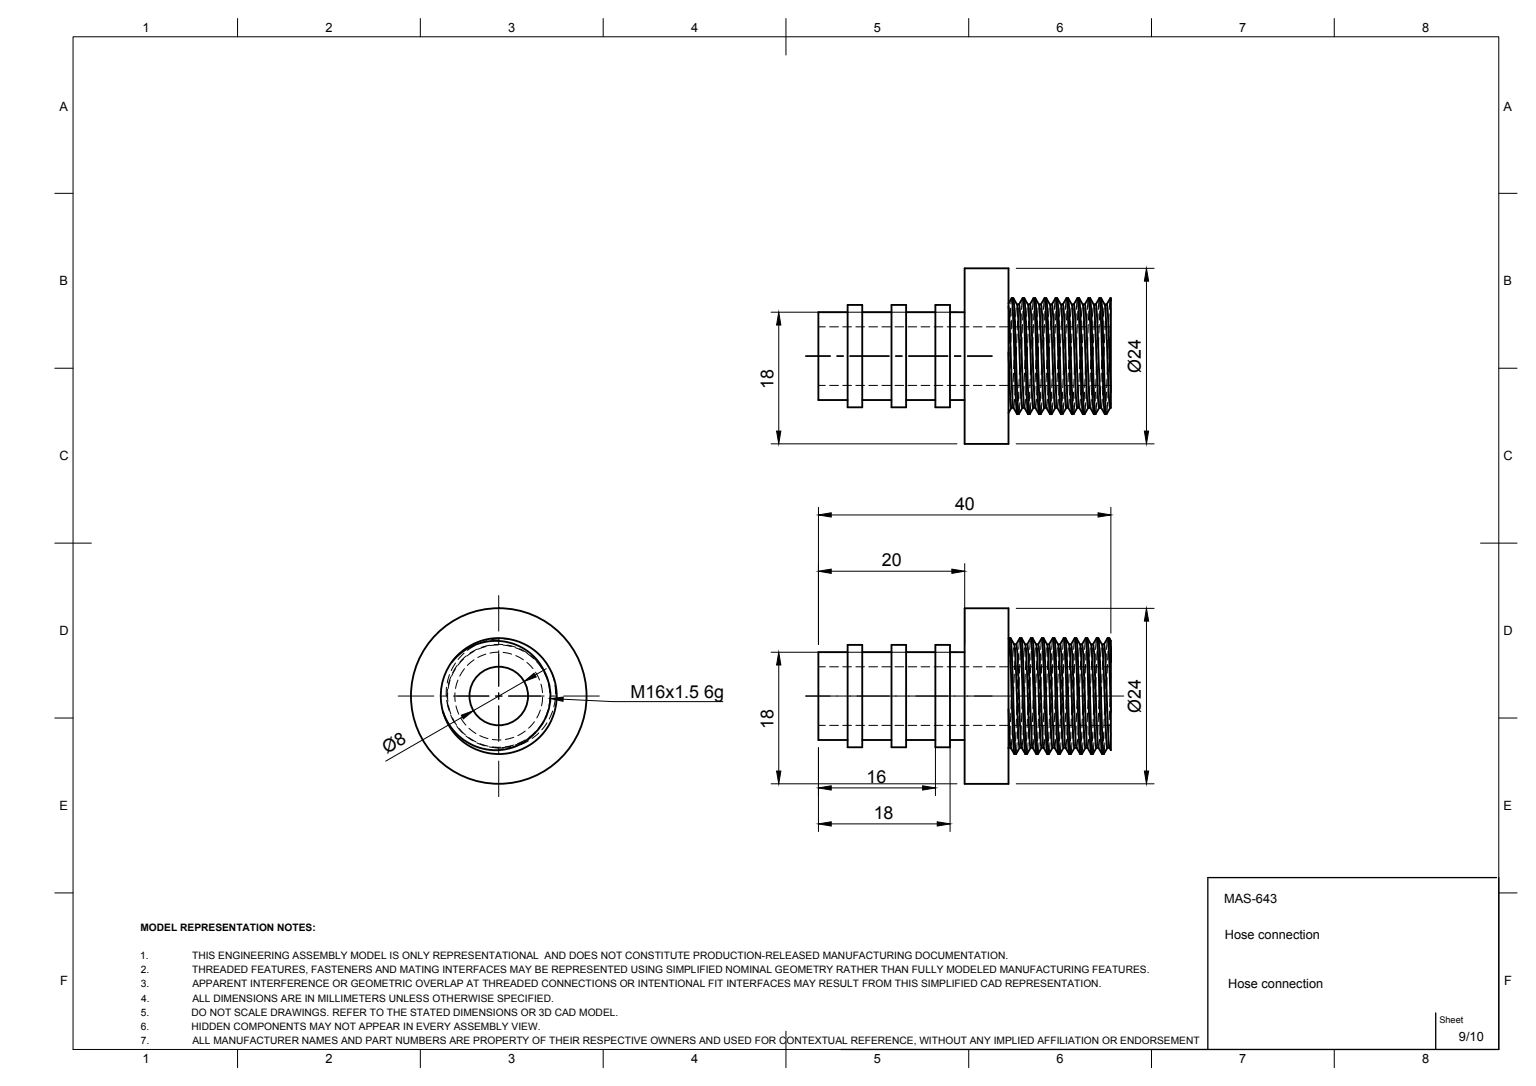
ISO-10303-21;
HEADER;
/* Generated by software containing ST-Developer
 * from STEP Tools, Inc. (www.steptools.com) 
 */

FILE_DESCRIPTION(
/* description */ ('Independent eighteen-tube parallel-flow evaporator geometry. Repeated
 machined headers and gasketed service covers, eighteen copper tubes, 
twenty-nine punched fins, threaded hose connections and bolted mountin
g feet. Native editable features and instanced parts. Braze details, w
orking fluid, pressure and thermal ratings require engineering selecti
on.'),
/* implementation_level */ '2;1');

FILE_NAME(
/* name */ 'Hose connection.step',
/* time_stamp */ '2026-11-08T20:53:59-08:00',
/* author */ (''),
/* organization */ (''),
/* preprocessor_version */ 'ST-DEVELOPER v20.2',
/* originating_system */ 'Autodesk Translation Framework v15.17.0.0',
/* authorisation */ '');

FILE_SCHEMA (('AUTOMOTIVE_DESIGN { 1 0 10303 214 3 1 1 }'));
ENDSEC;

DATA;
#10=MECHANICAL_DESIGN_GEOMETRIC_PRESENTATION_REPRESENTATION('',(#341),#42620);
#321=SHAPE_REPRESENTATION_RELATIONSHIP('SRR','None',#42731,#331);
#331=ADVANCED_BREP_SHAPE_REPRESENTATION('',(#351),#42618);
#341=STYLED_ITEM('',(#42787),#351);
#351=MANIFOLD_SOLID_BREP('Body1',#10391);
#475=FACE_BOUND('',#1791,.T.);
#476=FACE_BOUND('',#1793,.T.);
#477=FACE_BOUND('',#1797,.T.);
#478=FACE_BOUND('',#1799,.T.);
#479=FACE_BOUND('',#1803,.T.);
#480=FACE_BOUND('',#1805,.T.);
#481=FACE_BOUND('',#1810,.T.);
#482=FACE_BOUND('',#1812,.T.);
#483=FACE_BOUND('',#1815,.T.);
#484=FACE_BOUND('',#1818,.T.);
#567=PLANE('',#11185);
#568=PLANE('',#11188);
#569=PLANE('',#11194);
#570=PLANE('',#11196);
#571=PLANE('',#11202);
#572=PLANE('',#11204);
#573=PLANE('',#11212);
#574=PLANE('',#11214);
#575=PLANE('',#11218);
#576=PLANE('',#11221);
#601=B_SPLINE_SURFACE_WITH_KNOTS('',3,3,((#40929,#40930,#40931,#40932,#40933,
#40934,#40935,#40936,#40937,#40938,#40939,#40940,#40941,#40942,#40943,#40944,
#40945,#40946,#40947,#40948,#40949,#40950,#40951,#40952,#40953,#40954,#40955,
#40956,#40957,#40958,#40959,#40960,#40961,#40962,#40963,#40964,#40965,#40966,
#40967,#40968,#40969,#40970,#40971,#40972,#40973,#40974,#40975,#40976,#40977,
#40978,#40979,#40980,#40981,#40982,#40983,#40984,#40985,#40986,#40987,#40988,
#40989,#40990,#40991,#40992,#40993,#40994,#40995,#40996,#40997,#40998,#40999,
#41000,#41001,#41002,#41003,#41004,#41005,#41006,#41007,#41008,#41009,#41010,
#41011,#41012,#41013,#41014,#41015,#41016,#41017,#41018,#41019,#41020,#41021,
#41022,#41023,#41024,#41025,#41026,#41027,#41028,#41029,#41030,#41031,#41032,
#41033,#41034,#41035,#41036,#41037,#41038,#41039,#41040,#41041,#41042,#41043,
#41044,#41045,#41046,#41047,#41048,#41049,#41050,#41051,#41052,#41053),
(#41054,#41055,#41056,#41057,#41058,#41059,#41060,#41061,#41062,#41063,
#41064,#41065,#41066,#41067,#41068,#41069,#41070,#41071,#41072,#41073,#41074,
#41075,#41076,#41077,#41078,#41079,#41080,#41081,#41082,#41083,#41084,#41085,
#41086,#41087,#41088,#41089,#41090,#41091,#41092,#41093,#41094,#41095,#41096,
#41097,#41098,#41099,#41100,#41101,#41102,#41103,#41104,#41105,#41106,#41107,
#41108,#41109,#41110,#41111,#41112,#41113,#41114,#41115,#41116,#41117,#41118,
#41119,#41120,#41121,#41122,#41123,#41124,#41125,#41126,#41127,#41128,#41129,
#41130,#41131,#41132,#41133,#41134,#41135,#41136,#41137,#41138,#41139,#41140,
#41141,#41142,#41143,#41144,#41145,#41146,#41147,#41148,#41149,#41150,#41151,
#41152,#41153,#41154,#41155,#41156,#41157,#41158,#41159,#41160,#41161,#41162,
#41163,#41164,#41165,#41166,#41167,#41168,#41169,#41170,#41171,#41172,#41173,
#41174,#41175,#41176,#41177,#41178),(#41179,#41180,#41181,#41182,#41183,
#41184,#41185,#41186,#41187,#41188,#41189,#41190,#41191,#41192,#41193,#41194,
#41195,#41196,#41197,#41198,#41199,#41200,#41201,#41202,#41203,#41204,#41205,
#41206,#41207,#41208,#41209,#41210,#41211,#41212,#41213,#41214,#41215,#41216,
#41217,#41218,#41219,#41220,#41221,#41222,#41223,#41224,#41225,#41226,#41227,
#41228,#41229,#41230,#41231,#41232,#41233,#41234,#41235,#41236,#41237,#41238,
#41239,#41240,#41241,#41242,#41243,#41244,#41245,#41246,#41247,#41248,#41249,
#41250,#41251,#41252,#41253,#41254,#41255,#41256,#41257,#41258,#41259,#41260,
#41261,#41262,#41263,#41264,#41265,#41266,#41267,#41268,#41269,#41270,#41271,
#41272,#41273,#41274,#41275,#41276,#41277,#41278,#41279,#41280,#41281,#41282,
#41283,#41284,#41285,#41286,#41287,#41288,#41289,#41290,#41291,#41292,#41293,
#41294,#41295,#41296,#41297,#41298,#41299,#41300,#41301,#41302,#41303),
(#41304,#41305,#41306,#41307,#41308,#41309,#41310,#41311,#41312,#41313,
#41314,#41315,#41316,#41317,#41318,#41319,#41320,#41321,#41322,#41323,#41324,
#41325,#41326,#41327,#41328,#41329,#41330,#41331,#41332,#41333,#41334,#41335,
#41336,#41337,#41338,#41339,#41340,#41341,#41342,#41343,#41344,#41345,#41346,
#41347,#41348,#41349,#41350,#41351,#41352,#41353,#41354,#41355,#41356,#41357,
#41358,#41359,#41360,#41361,#41362,#41363,#41364,#41365,#41366,#41367,#41368,
#41369,#41370,#41371,#41372,#41373,#41374,#41375,#41376,#41377,#41378,#41379,
#41380,#41381,#41382,#41383,#41384,#41385,#41386,#41387,#41388,#41389,#41390,
#41391,#41392,#41393,#41394,#41395,#41396,#41397,#41398,#41399,#41400,#41401,
#41402,#41403,#41404,#41405,#41406,#41407,#41408,#41409,#41410,#41411,#41412,
#41413,#41414,#41415,#41416,#41417,#41418,#41419,#41420,#41421,#41422,#41423,
#41424,#41425,#41426,#41427,#41428)),.UNSPECIFIED.,.F.,.F.,.F.,(4,4),(4,
1,1,1,1,1,1,1,1,1,1,1,1,1,1,1,1,1,1,1,1,1,1,1,1,1,1,1,1,1,1,1,1,1,1,1,1,
1,1,1,1,1,1,1,1,1,1,1,1,1,1,1,1,1,1,1,1,1,1,1,1,1,1,1,1,1,1,1,1,1,1,1,1,
1,1,1,1,1,1,1,1,1,1,1,1,1,1,1,1,1,1,1,1,1,1,1,1,1,1,1,1,1,1,1,1,1,1,1,1,
1,1,1,1,1,1,1,1,1,1,1,1,1,4),(0.,0.0989001011121828),(8.30505915324874,
8.80271834784681,9.30037754244489,9.79803673704296,10.295695931641,10.7933551262391,
11.2910143208372,11.7886735154353,12.2863327100333,12.7839919046314,13.2816510992295,
13.7793102938275,14.2769694884256,14.7746286830237,15.2722878776218,15.7699470722198,
16.2676062668179,16.765265461416,17.2629246560141,17.7605838506121,18.2582430452102,
18.7559022398083,19.2535614344064,19.7512206290044,20.2488798236025,20.7465390182006,
21.2441982127987,21.7418574073967,22.2395166019948,22.7371757965929,23.2348349911909,
23.732494185789,24.2301533803871,24.7278125749852,25.2254717695832,25.7231309641813,
26.2207901587794,26.7184493533775,27.2161085479755,27.7137677425736,28.2114269371717,
28.7090861317698,29.2067453263678,29.7044045209659,30.202063715564,30.699722910162,
31.1973821047601,31.6950412993582,32.1927004939563,32.6903596885543,33.1880188831524,
33.6856780777505,34.1833372723486,34.6809964669466,35.1786556615447,35.6763148561428,
36.1739740507409,36.6716332453389,37.169292439937,37.6669516345351,38.1646108291331,
38.6622700237312,39.1599292183293,39.6575884129274,40.1552476075254,40.6529068021235,
41.1505659967216,41.6482251913197,42.1458843859177,42.6435435805158,43.1412027751139,
43.638861969712,44.13652116431,44.6341803589081,45.1318395535062,45.6294987481042,
46.1271579427023,46.6248171373004,47.1224763318985,47.6201355264965,48.1177947210946,
48.6154539156927,49.1131131102908,49.6107723048888,50.1084314994869,50.606090694085,
51.103749888683,51.6014090832811,52.0990682778792,52.5967274724773,53.0943866670753,
53.5920458616734,54.0897050562715,54.5873642508696,55.0850234454676,55.5826826400657,
56.0803418346638,56.5780010292619,57.0756602238599,57.573319418458,58.0709786130561,
58.5686378076541,59.0662970022522,59.5639561968503,60.0616153914484,60.5592745860464,
61.0569337806445,61.5545929752426,62.0522521698407,62.5499113644387,63.0475705590368,
63.5452297536349,64.042888948233,64.540548142831,65.0382073374291,65.5358665320272,
66.0335257266252,66.5311849212233,67.0288441158214,67.5265033104195,68.0241625050175,
68.5218216996156,69.0194808942137),.UNSPECIFIED.);
#602=B_SPLINE_SURFACE_WITH_KNOTS('',3,3,((#41703,#41704,#41705,#41706,#41707,
#41708,#41709,#41710,#41711,#41712,#41713,#41714,#41715,#41716,#41717,#41718,
#41719,#41720,#41721,#41722,#41723,#41724,#41725,#41726,#41727,#41728,#41729,
#41730,#41731,#41732,#41733,#41734,#41735,#41736,#41737,#41738,#41739,#41740,
#41741,#41742,#41743,#41744,#41745,#41746,#41747,#41748,#41749,#41750,#41751,
#41752,#41753,#41754,#41755,#41756,#41757,#41758,#41759,#41760,#41761,#41762,
#41763,#41764,#41765,#41766,#41767,#41768,#41769,#41770,#41771,#41772,#41773,
#41774,#41775,#41776,#41777,#41778,#41779,#41780,#41781,#41782,#41783,#41784,
#41785,#41786,#41787,#41788,#41789,#41790,#41791,#41792,#41793,#41794,#41795,
#41796,#41797,#41798,#41799,#41800,#41801,#41802,#41803,#41804,#41805,#41806,
#41807,#41808,#41809,#41810,#41811,#41812,#41813,#41814,#41815,#41816,#41817,
#41818,#41819,#41820,#41821,#41822,#41823,#41824,#41825,#41826,#41827),
(#41828,#41829,#41830,#41831,#41832,#41833,#41834,#41835,#41836,#41837,
#41838,#41839,#41840,#41841,#41842,#41843,#41844,#41845,#41846,#41847,#41848,
#41849,#41850,#41851,#41852,#41853,#41854,#41855,#41856,#41857,#41858,#41859,
#41860,#41861,#41862,#41863,#41864,#41865,#41866,#41867,#41868,#41869,#41870,
#41871,#41872,#41873,#41874,#41875,#41876,#41877,#41878,#41879,#41880,#41881,
#41882,#41883,#41884,#41885,#41886,#41887,#41888,#41889,#41890,#41891,#41892,
#41893,#41894,#41895,#41896,#41897,#41898,#41899,#41900,#41901,#41902,#41903,
#41904,#41905,#41906,#41907,#41908,#41909,#41910,#41911,#41912,#41913,#41914,
#41915,#41916,#41917,#41918,#41919,#41920,#41921,#41922,#41923,#41924,#41925,
#41926,#41927,#41928,#41929,#41930,#41931,#41932,#41933,#41934,#41935,#41936,
#41937,#41938,#41939,#41940,#41941,#41942,#41943,#41944,#41945,#41946,#41947,
#41948,#41949,#41950,#41951,#41952),(#41953,#41954,#41955,#41956,#41957,
#41958,#41959,#41960,#41961,#41962,#41963,#41964,#41965,#41966,#41967,#41968,
#41969,#41970,#41971,#41972,#41973,#41974,#41975,#41976,#41977,#41978,#41979,
#41980,#41981,#41982,#41983,#41984,#41985,#41986,#41987,#41988,#41989,#41990,
#41991,#41992,#41993,#41994,#41995,#41996,#41997,#41998,#41999,#42000,#42001,
#42002,#42003,#42004,#42005,#42006,#42007,#42008,#42009,#42010,#42011,#42012,
#42013,#42014,#42015,#42016,#42017,#42018,#42019,#42020,#42021,#42022,#42023,
#42024,#42025,#42026,#42027,#42028,#42029,#42030,#42031,#42032,#42033,#42034,
#42035,#42036,#42037,#42038,#42039,#42040,#42041,#42042,#42043,#42044,#42045,
#42046,#42047,#42048,#42049,#42050,#42051,#42052,#42053,#42054,#42055,#42056,
#42057,#42058,#42059,#42060,#42061,#42062,#42063,#42064,#42065,#42066,#42067,
#42068,#42069,#42070,#42071,#42072,#42073,#42074,#42075,#42076,#42077),
(#42078,#42079,#42080,#42081,#42082,#42083,#42084,#42085,#42086,#42087,
#42088,#42089,#42090,#42091,#42092,#42093,#42094,#42095,#42096,#42097,#42098,
#42099,#42100,#42101,#42102,#42103,#42104,#42105,#42106,#42107,#42108,#42109,
#42110,#42111,#42112,#42113,#42114,#42115,#42116,#42117,#42118,#42119,#42120,
#42121,#42122,#42123,#42124,#42125,#42126,#42127,#42128,#42129,#42130,#42131,
#42132,#42133,#42134,#42135,#42136,#42137,#42138,#42139,#42140,#42141,#42142,
#42143,#42144,#42145,#42146,#42147,#42148,#42149,#42150,#42151,#42152,#42153,
#42154,#42155,#42156,#42157,#42158,#42159,#42160,#42161,#42162,#42163,#42164,
#42165,#42166,#42167,#42168,#42169,#42170,#42171,#42172,#42173,#42174,#42175,
#42176,#42177,#42178,#42179,#42180,#42181,#42182,#42183,#42184,#42185,#42186,
#42187,#42188,#42189,#42190,#42191,#42192,#42193,#42194,#42195,#42196,#42197,
#42198,#42199,#42200,#42201,#42202)),.UNSPECIFIED.,.F.,.F.,.F.,(4,4),(4,
1,1,1,1,1,1,1,1,1,1,1,1,1,1,1,1,1,1,1,1,1,1,1,1,1,1,1,1,1,1,1,1,1,1,1,1,
1,1,1,1,1,1,1,1,1,1,1,1,1,1,1,1,1,1,1,1,1,1,1,1,1,1,1,1,1,1,1,1,1,1,1,1,
1,1,1,1,1,1,1,1,1,1,1,1,1,1,1,1,1,1,1,1,1,1,1,1,1,1,1,1,1,1,1,1,1,1,1,1,
1,1,1,1,1,1,1,1,1,1,1,1,1,4),(0.,0.0989001011121828),(11.6147305479242,
12.1123897425223,12.6100489371204,13.1077081317185,13.6053673263165,14.1030265209146,
14.6006857155127,15.0983449101107,15.5960041047088,16.0936632993069,16.591322493905,
17.088981688503,17.5866408831011,18.0843000776992,18.5819592722973,19.0796184668953,
19.5772776614934,20.0749368560915,20.5725960506896,21.0702552452876,21.5679144398857,
22.0655736344838,22.5632328290818,23.0608920236799,23.558551218278,24.0562104128761,
24.5538696074741,25.0515288020722,25.5491879966703,26.0468471912684,26.5445063858664,
27.0421655804645,27.5398247750626,28.0374839696607,28.5351431642587,29.0328023588568,
29.5304615534549,30.0281207480529,30.525779942651,31.0234391372491,31.5210983318472,
32.0187575264452,32.5164167210433,33.0140759156414,33.5117351102395,34.0093943048375,
34.5070534994356,35.0047126940337,35.5023718886318,36.0000310832298,36.4976902778279,
36.995349472426,37.4930086670241,37.9906678616221,38.4883270562202,38.9859862508183,
39.4836454454163,39.9813046400144,40.4789638346125,40.9766230292106,41.4742822238086,
41.9719414184067,42.4696006130048,42.9672598076029,43.4649190022009,43.962578196799,
44.4602373913971,44.9578965859952,45.4555557805932,45.9532149751913,46.4508741697894,
46.9485333643874,47.4461925589855,47.9438517535836,48.4415109481817,48.9391701427797,
49.4368293373778,49.9344885319759,50.432147726574,50.929806921172,51.4274661157701,
51.9251253103682,52.4227845049663,52.9204436995643,53.4181028941624,53.9157620887605,
54.4134212833585,54.9110804779566,55.4087396725547,55.9063988671528,56.4040580617508,
56.9017172563489,57.399376450947,57.8970356455451,58.3946948401431,58.8923540347412,
59.3900132293393,59.8876724239374,60.3853316185354,60.8829908131335,61.3806500077316,
61.8783092023296,62.3759683969277,62.8736275915258,63.3712867861239,63.8689459807219,
64.36660517532,64.8642643699181,65.3619235645162,65.8595827591142,66.3572419537123,
66.8549011483104,67.3525603429085,67.8502195375065,68.3478787321046,68.8455379267027,
69.3431971213007,69.8408563158988,70.3385155104969,70.836174705095,71.333833899693,
71.8314930942911,72.3291522888892),.UNSPECIFIED.);
#1101=FACE_OUTER_BOUND('',#1767,.T.);
#1102=FACE_OUTER_BOUND('',#1768,.T.);
#1103=FACE_OUTER_BOUND('',#1769,.T.);
#1104=FACE_OUTER_BOUND('',#1770,.T.);
#1105=FACE_OUTER_BOUND('',#1771,.T.);
#1106=FACE_OUTER_BOUND('',#1772,.T.);
#1107=FACE_OUTER_BOUND('',#1773,.T.);
#1108=FACE_OUTER_BOUND('',#1774,.T.);
#1109=FACE_OUTER_BOUND('',#1775,.T.);
#1110=FACE_OUTER_BOUND('',#1776,.T.);
#1111=FACE_OUTER_BOUND('',#1777,.T.);
#1112=FACE_OUTER_BOUND('',#1778,.T.);
#1113=FACE_OUTER_BOUND('',#1779,.T.);
#1114=FACE_OUTER_BOUND('',#1780,.T.);
#1115=FACE_OUTER_BOUND('',#1781,.T.);
#1116=FACE_OUTER_BOUND('',#1782,.T.);
#1117=FACE_OUTER_BOUND('',#1783,.T.);
#1118=FACE_OUTER_BOUND('',#1784,.T.);
#1119=FACE_OUTER_BOUND('',#1785,.T.);
#1120=FACE_OUTER_BOUND('',#1786,.T.);
#1121=FACE_OUTER_BOUND('',#1787,.T.);
#1122=FACE_OUTER_BOUND('',#1788,.T.);
#1123=FACE_OUTER_BOUND('',#1789,.T.);
#1124=FACE_OUTER_BOUND('',#1790,.T.);
#1125=FACE_OUTER_BOUND('',#1792,.T.);
#1126=FACE_OUTER_BOUND('',#1794,.T.);
#1127=FACE_OUTER_BOUND('',#1795,.T.);
#1128=FACE_OUTER_BOUND('',#1796,.T.);
#1129=FACE_OUTER_BOUND('',#1798,.T.);
#1130=FACE_OUTER_BOUND('',#1800,.T.);
#1131=FACE_OUTER_BOUND('',#1801,.T.);
#1132=FACE_OUTER_BOUND('',#1802,.T.);
#1133=FACE_OUTER_BOUND('',#1804,.T.);
#1134=FACE_OUTER_BOUND('',#1806,.T.);
#1135=FACE_OUTER_BOUND('',#1807,.T.);
#1136=FACE_OUTER_BOUND('',#1808,.T.);
#1137=FACE_OUTER_BOUND('',#1809,.T.);
#1138=FACE_OUTER_BOUND('',#1811,.T.);
#1139=FACE_OUTER_BOUND('',#1813,.T.);
#1140=FACE_OUTER_BOUND('',#1814,.T.);
#1141=FACE_OUTER_BOUND('',#1816,.T.);
#1142=FACE_OUTER_BOUND('',#1817,.T.);
#1767=EDGE_LOOP('',(#9209,#9210,#9211,#9212));
#1768=EDGE_LOOP('',(#9213,#9214,#9215,#9216));
#1769=EDGE_LOOP('',(#9217,#9218,#9219,#9220));
#1770=EDGE_LOOP('',(#9221,#9222,#9223,#9224));
#1771=EDGE_LOOP('',(#9225,#9226,#9227,#9228));
#1772=EDGE_LOOP('',(#9229,#9230,#9231,#9232));
#1773=EDGE_LOOP('',(#9233,#9234,#9235,#9236));
#1774=EDGE_LOOP('',(#9237,#9238,#9239,#9240));
#1775=EDGE_LOOP('',(#9241,#9242,#9243,#9244));
#1776=EDGE_LOOP('',(#9245,#9246,#9247,#9248));
#1777=EDGE_LOOP('',(#9249,#9250,#9251,#9252));
#1778=EDGE_LOOP('',(#9253,#9254,#9255,#9256));
#1779=EDGE_LOOP('',(#9257,#9258,#9259,#9260));
#1780=EDGE_LOOP('',(#9261,#9262,#9263,#9264));
#1781=EDGE_LOOP('',(#9265,#9266,#9267,#9268));
#1782=EDGE_LOOP('',(#9269,#9270,#9271,#9272));
#1783=EDGE_LOOP('',(#9273,#9274,#9275,#9276));
#1784=EDGE_LOOP('',(#9277,#9278,#9279,#9280));
#1785=EDGE_LOOP('',(#9281,#9282,#9283,#9284));
#1786=EDGE_LOOP('',(#9285,#9286,#9287,#9288,#9289,#9290,#9291,#9292,#9293,
#9294,#9295,#9296,#9297,#9298,#9299,#9300,#9301,#9302,#9303,#9304,#9305,
#9306,#9307));
#1787=EDGE_LOOP('',(#9308,#9309,#9310,#9311));
#1788=EDGE_LOOP('',(#9312,#9313,#9314,#9315,#9316,#9317,#9318,#9319,#9320,
#9321,#9322,#9323,#9324,#9325,#9326,#9327,#9328,#9329,#9330,#9331,#9332,
#9333,#9334));
#1789=EDGE_LOOP('',(#9335,#9336,#9337,#9338));
#1790=EDGE_LOOP('',(#9339));
#1791=EDGE_LOOP('',(#9340));
#1792=EDGE_LOOP('',(#9341));
#1793=EDGE_LOOP('',(#9342));
#1794=EDGE_LOOP('',(#9343,#9344,#9345,#9346));
#1795=EDGE_LOOP('',(#9347,#9348,#9349,#9350));
#1796=EDGE_LOOP('',(#9351));
#1797=EDGE_LOOP('',(#9352));
#1798=EDGE_LOOP('',(#9353));
#1799=EDGE_LOOP('',(#9354));
#1800=EDGE_LOOP('',(#9355,#9356,#9357,#9358));
#1801=EDGE_LOOP('',(#9359,#9360,#9361,#9362));
#1802=EDGE_LOOP('',(#9363));
#1803=EDGE_LOOP('',(#9364));
#1804=EDGE_LOOP('',(#9365));
#1805=EDGE_LOOP('',(#9366));
#1806=EDGE_LOOP('',(#9367,#9368,#9369,#9370));
#1807=EDGE_LOOP('',(#9371,#9372,#9373,#9374));
#1808=EDGE_LOOP('',(#9375,#9376,#9377,#9378));
#1809=EDGE_LOOP('',(#9379));
#1810=EDGE_LOOP('',(#9380));
#1811=EDGE_LOOP('',(#9381));
#1812=EDGE_LOOP('',(#9382,#9383,#9384,#9385));
#1813=EDGE_LOOP('',(#9386,#9387,#9388,#9389));
#1814=EDGE_LOOP('',(#9390));
#1815=EDGE_LOOP('',(#9391));
#1816=EDGE_LOOP('',(#9392,#9393,#9394,#9395));
#1817=EDGE_LOOP('',(#9396,#9397,#9398,#9399));
#1818=EDGE_LOOP('',(#9400));
#1995=CIRCLE('',#11161,7.925);
#1996=CIRCLE('',#11172,7.0685);
#1997=CIRCLE('',#11182,7.0685);
#1998=CIRCLE('',#11184,7.925);
#1999=CIRCLE('',#11186,7.);
#2000=CIRCLE('',#11187,6.);
#2001=CIRCLE('',#11189,7.);
#2002=CIRCLE('',#11190,6.);
#2003=CIRCLE('',#11193,6.);
#2004=CIRCLE('',#11195,7.);
#2005=CIRCLE('',#11197,7.);
#2006=CIRCLE('',#11198,6.);
#2007=CIRCLE('',#11201,6.);
#2008=CIRCLE('',#11203,7.);
#2009=CIRCLE('',#11205,7.);
#2010=CIRCLE('',#11206,6.);
#2011=CIRCLE('',#11209,6.);
#2012=CIRCLE('',#11211,6.);
#2013=CIRCLE('',#11213,4.);
#2014=CIRCLE('',#11215,12.);
#2015=CIRCLE('',#11217,12.);
#2016=CIRCLE('',#11220,4.);
#2753=B_SPLINE_CURVE_WITH_KNOTS('',3,(#39788,#39789,#39790,#39791,#39792,
#39793,#39794,#39795,#39796,#39797,#39798,#39799,#39800,#39801,#39802,#39803),
 .UNSPECIFIED.,.F.,.F.,(4,3,3,3,3,4),(-4.09323272002468,-3.98127355678459,
-3.48361436218651,-2.98595516758844,-2.48829597299037,-2.07135887395548),
 .UNSPECIFIED.);
#2754=B_SPLINE_CURVE_WITH_KNOTS('',3,(#39806,#39807,#39808,#39809,#39810,
#39811,#39812,#39813,#39814,#39815),.UNSPECIFIED.,.F.,.F.,(4,3,3,4),(0.,
0.497659194598067,0.995318389196143,1.11971880752056),.UNSPECIFIED.);
#2755=B_SPLINE_CURVE_WITH_KNOTS('',3,(#39820,#39821,#39822,#39823,#39824,
#39825,#39826,#39827,#39828,#39829,#39830,#39831,#39832,#39833,#39834,#39835,
#39836,#39837,#39838,#39839,#39840,#39841,#39842,#39843,#39844,#39845,#39846,
#39847,#39848,#39849,#39850,#39851,#39852,#39853,#39854,#39855,#39856,#39857,
#39858,#39859),.UNSPECIFIED.,.F.,.F.,(4,3,3,3,3,3,3,3,3,3,3,3,3,4),(-10.3764180272043,
-9.95318389196147,-9.45552469736339,-8.95786550276532,-8.46020630816725,
-7.96254711356918,-7.4648879189711,-6.96722872437303,-6.46956952977495,
-5.97191033517688,-5.47425114057881,-4.97659194598073,-4.47893275138266,
-4.09323272002468),.UNSPECIFIED.);
#2756=B_SPLINE_CURVE_WITH_KNOTS('',3,(#39860,#39861,#39862,#39863,#39864,
#39865,#39866,#39867,#39868,#39869,#39870,#39871,#39872,#39873,#39874,#39875,
#39876,#39877,#39878,#39879,#39880,#39881,#39882,#39883,#39884,#39885,#39886,
#39887,#39888,#39889,#39890,#39891,#39892,#39893,#39894,#39895,#39896,#39897,
#39898,#39899),.UNSPECIFIED.,.F.,.F.,(4,3,3,3,3,3,3,3,3,3,3,3,3,4),(1.11971880752056,
1.49297758379422,1.99063677839229,2.48829597299036,2.98595516758844,3.48361436218651,
3.98127355678458,4.47893275138265,4.97659194598073,5.4742511405788,5.97191033517688,
6.46956952977495,6.96722872437302,7.40290411470015),.UNSPECIFIED.);
#2757=B_SPLINE_CURVE_WITH_KNOTS('',3,(#39904,#39905,#39906,#39907,#39908,
#39909,#39910,#39911,#39912,#39913,#39914,#39915,#39916,#39917,#39918,#39919,
#39920,#39921,#39922,#39923,#39924,#39925,#39926,#39927,#39928,#39929,#39930,
#39931,#39932,#39933,#39934,#39935,#39936,#39937,#39938,#39939,#39940,#39941,
#39942,#39943,#39944,#39945,#39946),.UNSPECIFIED.,.F.,.F.,(4,3,3,3,3,3,
3,3,3,3,3,3,3,3,4),(-16.6596033343839,-16.4227534217364,-15.9250942271383,
-15.4274350325403,-14.9297758379422,-14.4321166433441,-13.9344574487461,
-13.436798254148,-12.9391390595499,-12.4414798649518,-11.9438206703538,
-11.4461614757557,-10.9485022811576,-10.4508430865595,-10.3764180272043),
 .UNSPECIFIED.);
#2758=B_SPLINE_CURVE_WITH_KNOTS('',3,(#39947,#39948,#39949,#39950,#39951,
#39952,#39953,#39954,#39955,#39956,#39957,#39958,#39959,#39960,#39961,#39962,
#39963,#39964,#39965,#39966,#39967,#39968,#39969,#39970,#39971,#39972,#39973,
#39974,#39975,#39976,#39977,#39978,#39979,#39980,#39981,#39982,#39983,#39984,
#39985,#39986,#39987,#39988,#39989),.UNSPECIFIED.,.F.,.F.,(4,3,3,3,3,3,
3,3,3,3,3,3,3,3,4),(7.40290411470015,7.4648879189711,7.96254711356917,8.46020630816724,
8.95786550276532,9.45552469736339,9.95318389196146,10.4508430865595,10.9485022811576,
11.4461614757557,11.9438206703538,12.4414798649518,12.9391390595499,13.436798254148,
13.6860894218797),.UNSPECIFIED.);
#2759=B_SPLINE_CURVE_WITH_KNOTS('',3,(#39994,#39995,#39996,#39997,#39998,
#39999,#40000,#40001,#40002,#40003,#40004,#40005,#40006,#40007,#40008,#40009,
#40010,#40011,#40012,#40013,#40014,#40015,#40016,#40017,#40018,#40019,#40020,
#40021,#40022,#40023,#40024,#40025,#40026,#40027,#40028,#40029,#40030,#40031,
#40032,#40033,#40034,#40035,#40036),.UNSPECIFIED.,.F.,.F.,(4,3,3,3,3,3,
3,3,3,3,3,3,3,3,4),(-22.9427886415634,-22.8923229515114,-22.3946637569133,
-21.8970045623152,-21.3993453677171,-20.9016861731191,-20.404026978521,
-19.9063677839229,-19.4087085893249,-18.9110493947268,-18.4133902001287,
-17.9157310055306,-17.4180718109326,-16.9204126163345,-16.6596033343839),
 .UNSPECIFIED.);
#2760=B_SPLINE_CURVE_WITH_KNOTS('',3,(#40037,#40038,#40039,#40040,#40041,
#40042,#40043,#40044,#40045,#40046,#40047,#40048,#40049,#40050,#40051,#40052,
#40053,#40054,#40055,#40056,#40057,#40058,#40059,#40060,#40061,#40062,#40063,
#40064,#40065,#40066,#40067,#40068,#40069,#40070,#40071,#40072,#40073,#40074,
#40075,#40076,#40077,#40078,#40079),.UNSPECIFIED.,.F.,.F.,(4,3,3,3,3,3,
3,3,3,3,3,3,3,3,4),(13.6860894218797,13.934457448746,14.4321166433441,14.9297758379422,
15.4274350325403,15.9250942271383,16.4227534217364,16.9204126163345,17.4180718109326,
17.9157310055306,18.4133902001287,18.9110493947268,19.4087085893249,19.9063677839229,
19.9692747290593),.UNSPECIFIED.);
#2761=B_SPLINE_CURVE_WITH_KNOTS('',3,(#40084,#40085,#40086,#40087,#40088,
#40089,#40090,#40091,#40092,#40093,#40094,#40095,#40096,#40097,#40098,#40099,
#40100,#40101,#40102,#40103,#40104,#40105,#40106,#40107,#40108,#40109,#40110,
#40111,#40112,#40113,#40114,#40115,#40116,#40117,#40118,#40119,#40120,#40121,
#40122,#40123),.UNSPECIFIED.,.F.,.F.,(4,3,3,3,3,3,3,3,3,3,3,3,3,4),(-29.225973948743,
-28.8642332866883,-28.3665740920902,-27.8689148974921,-27.371255702894,
-26.873596508296,-26.3759373136979,-25.8782781190998,-25.3806189245017,
-24.8829597299037,-24.3853005353056,-23.8876413407075,-23.3899821461094,
-22.9427886415634),.UNSPECIFIED.);
#2762=B_SPLINE_CURVE_WITH_KNOTS('',3,(#40124,#40125,#40126,#40127,#40128,
#40129,#40130,#40131,#40132,#40133,#40134,#40135,#40136,#40137,#40138,#40139,
#40140,#40141,#40142,#40143,#40144,#40145,#40146,#40147,#40148,#40149,#40150,
#40151,#40152,#40153,#40154,#40155,#40156,#40157,#40158,#40159,#40160,#40161,
#40162,#40163),.UNSPECIFIED.,.F.,.F.,(4,3,3,3,3,3,3,3,3,3,3,3,3,4),(19.9692747290593,
20.404026978521,20.9016861731191,21.3993453677172,21.8970045623152,22.3946637569133,
22.8923229515114,23.3899821461095,23.8876413407075,24.3853005353056,24.8829597299037,
25.3806189245017,25.8782781190998,26.2524600362389),.UNSPECIFIED.);
#2763=B_SPLINE_CURVE_WITH_KNOTS('',3,(#40168,#40169,#40170,#40171,#40172,
#40173,#40174,#40175,#40176,#40177,#40178,#40179,#40180,#40181,#40182,#40183,
#40184,#40185,#40186,#40187,#40188,#40189,#40190,#40191,#40192,#40193,#40194,
#40195,#40196,#40197,#40198,#40199,#40200,#40201,#40202,#40203,#40204,#40205,
#40206,#40207,#40208,#40209,#40210),.UNSPECIFIED.,.F.,.F.,(4,3,3,3,3,3,
3,3,3,3,3,3,3,3,4),(-35.5091592559226,-35.3338028164632,-34.8361436218651,
-34.3384844272671,-33.840825232669,-33.3431660380709,-32.8455068434729,
-32.3478476488748,-31.8501884542767,-31.3525292596786,-30.8548700650806,
-30.3572108704825,-29.8595516758844,-29.3618924812863,-29.225973948743),
 .UNSPECIFIED.);
#2764=B_SPLINE_CURVE_WITH_KNOTS('',3,(#40211,#40212,#40213,#40214,#40215,
#40216,#40217,#40218,#40219,#40220,#40221,#40222,#40223,#40224,#40225,#40226,
#40227,#40228,#40229,#40230,#40231,#40232,#40233,#40234,#40235,#40236,#40237,
#40238,#40239,#40240,#40241,#40242,#40243,#40244,#40245,#40246,#40247,#40248,
#40249,#40250,#40251,#40252,#40253),.UNSPECIFIED.,.F.,.F.,(4,3,3,3,3,3,
3,3,3,3,3,3,3,3,4),(26.2524600362389,26.3759373136979,26.873596508296,27.371255702894,
27.8689148974921,28.3665740920902,28.8642332866883,29.3618924812863,29.8595516758844,
30.3572108704825,30.8548700650806,31.3525292596786,31.8501884542767,32.3478476488748,
32.5356453434185),.UNSPECIFIED.);
#2765=B_SPLINE_CURVE_WITH_KNOTS('',3,(#40258,#40259,#40260,#40261,#40262,
#40263,#40264,#40265,#40266,#40267,#40268,#40269,#40270,#40271,#40272,#40273,
#40274,#40275,#40276,#40277,#40278,#40279,#40280,#40281,#40282,#40283,#40284,
#40285,#40286,#40287,#40288,#40289,#40290,#40291,#40292,#40293,#40294,#40295,
#40296,#40297),.UNSPECIFIED.,.F.,.F.,(4,3,3,3,3,3,3,3,3,3,3,3,3,4),(-41.7923445631022,
-41.3057131516401,-40.808053957042,-40.3103947624439,-39.8127355678459,
-39.3150763732478,-38.8174171786497,-38.3197579840517,-37.8220987894536,
-37.3244395948555,-36.8267804002574,-36.3291212056594,-35.8314620110613,
-35.5091592559226),.UNSPECIFIED.);
#2766=B_SPLINE_CURVE_WITH_KNOTS('',3,(#40298,#40299,#40300,#40301,#40302,
#40303,#40304,#40305,#40306,#40307,#40308,#40309,#40310,#40311,#40312,#40313,
#40314,#40315,#40316,#40317,#40318,#40319,#40320,#40321,#40322,#40323,#40324,
#40325,#40326,#40327,#40328,#40329,#40330,#40331,#40332,#40333,#40334,#40335,
#40336,#40337,#40338,#40339,#40340),.UNSPECIFIED.,.F.,.F.,(4,3,3,3,3,3,
3,3,3,3,3,3,3,3,4),(32.5356453434185,32.8455068434728,33.3431660380709,
33.840825232669,34.3384844272671,34.8361436218651,35.3338028164632,35.8314620110613,
36.3291212056594,36.8267804002574,37.3244395948555,37.8220987894536,38.3197579840516,
38.8174171786497,38.8188306505981),.UNSPECIFIED.);
#2767=B_SPLINE_CURVE_WITH_KNOTS('',3,(#40345,#40346,#40347,#40348,#40349,
#40350,#40351,#40352,#40353,#40354,#40355,#40356,#40357,#40358,#40359,#40360,
#40361,#40362,#40363,#40364,#40365,#40366,#40367,#40368,#40369,#40370,#40371,
#40372,#40373,#40374,#40375,#40376,#40377,#40378,#40379,#40380,#40381,#40382,
#40383,#40384,#40385,#40386,#40387),.UNSPECIFIED.,.F.,.F.,(4,3,3,3,3,3,
3,3,3,3,3,3,3,3,4),(-48.0755298702818,-47.7752826814151,-47.277623486817,
-46.7799642922189,-46.2823050976208,-45.7846459030228,-45.2869867084247,
-44.7893275138266,-44.2916683192285,-43.7940091246305,-43.2963499300324,
-42.7986907354343,-42.3010315408362,-41.8033723462382,-41.7923445631022),
 .UNSPECIFIED.);
#2768=B_SPLINE_CURVE_WITH_KNOTS('',3,(#40388,#40389,#40390,#40391,#40392,
#40393,#40394,#40395,#40396,#40397,#40398,#40399,#40400,#40401,#40402,#40403,
#40404,#40405,#40406,#40407,#40408,#40409,#40410,#40411,#40412,#40413,#40414,
#40415,#40416,#40417,#40418,#40419,#40420,#40421,#40422,#40423,#40424,#40425,
#40426,#40427),.UNSPECIFIED.,.F.,.F.,(4,3,3,3,3,3,3,3,3,3,3,3,3,4),(38.8188306505981,
39.3150763732478,39.8127355678459,40.3103947624439,40.808053957042,41.3057131516401,
41.8033723462382,42.3010315408362,42.7986907354343,43.2963499300324,43.7940091246304,
44.2916683192285,44.7893275138266,45.1020159577777),.UNSPECIFIED.);
#2769=B_SPLINE_CURVE_WITH_KNOTS('',3,(#40432,#40433,#40434,#40435,#40436,
#40437,#40438,#40439,#40440,#40441,#40442,#40443,#40444,#40445,#40446,#40447,
#40448,#40449,#40450,#40451,#40452,#40453,#40454,#40455,#40456,#40457,#40458,
#40459,#40460,#40461,#40462,#40463,#40464,#40465,#40466,#40467,#40468,#40469,
#40470,#40471,#40472,#40473,#40474),.UNSPECIFIED.,.F.,.F.,(4,3,3,3,3,3,
3,3,3,3,3,3,3,3,4),(-54.3587151774614,-54.24485221119,-53.7471930165919,
-53.2495338219939,-52.7518746273958,-52.2542154327977,-51.7565562381996,
-51.2588970436016,-50.7612378490035,-50.2635786544054,-49.7659194598073,
-49.2682602652093,-48.7706010706112,-48.2729418760131,-48.0755298702818),
 .UNSPECIFIED.);
#2770=B_SPLINE_CURVE_WITH_KNOTS('',3,(#40475,#40476,#40477,#40478,#40479,
#40480,#40481,#40482,#40483,#40484,#40485,#40486,#40487,#40488,#40489,#40490,
#40491,#40492,#40493,#40494,#40495,#40496,#40497,#40498,#40499,#40500,#40501,
#40502,#40503,#40504,#40505,#40506,#40507,#40508,#40509,#40510,#40511,#40512,
#40513,#40514,#40515,#40516,#40517),.UNSPECIFIED.,.F.,.F.,(4,3,3,3,3,3,
3,3,3,3,3,3,3,3,4),(45.1020159577777,45.2869867084247,45.7846459030227,
46.2823050976208,46.7799642922189,47.277623486817,47.775282681415,48.2729418760131,
48.7706010706112,49.2682602652093,49.7659194598073,50.2635786544054,50.7612378490035,
51.2588970436016,51.3852012649573),.UNSPECIFIED.);
#2771=B_SPLINE_CURVE_WITH_KNOTS('',3,(#40522,#40523,#40524,#40525,#40526,
#40527,#40528,#40529,#40530,#40531,#40532,#40533,#40534,#40535,#40536,#40537,
#40538,#40539,#40540,#40541,#40542,#40543,#40544,#40545,#40546,#40547,#40548,
#40549,#40550,#40551,#40552,#40553,#40554,#40555,#40556,#40557,#40558,#40559,
#40560,#40561),.UNSPECIFIED.,.F.,.F.,(4,3,3,3,3,3,3,3,3,3,3,3,3,4),(-60.641900484641,
-60.2167625463669,-59.7191033517688,-59.2214441571707,-58.7237849625727,
-58.2261257679746,-57.7284665733765,-57.2308073787784,-56.7331481841804,
-56.2354889895823,-55.7378297949842,-55.2401706003861,-54.7425114057881,
-54.3587151774614),.UNSPECIFIED.);
#2772=B_SPLINE_CURVE_WITH_KNOTS('',3,(#40562,#40563,#40564,#40565,#40566,
#40567,#40568,#40569,#40570,#40571,#40572,#40573,#40574,#40575,#40576,#40577,
#40578,#40579,#40580,#40581,#40582,#40583,#40584,#40585,#40586,#40587,#40588,
#40589,#40590,#40591,#40592,#40593,#40594,#40595,#40596,#40597,#40598,#40599,
#40600,#40601),.UNSPECIFIED.,.F.,.F.,(4,3,3,3,3,3,3,3,3,3,3,3,3,4),(51.3852012649573,
51.7565562381996,52.2542154327977,52.7518746273958,53.2495338219938,53.7471930165919,
54.24485221119,54.7425114057881,55.2401706003861,55.7378297949842,56.2354889895823,
56.7331481841804,57.2308073787784,57.6683865721369),.UNSPECIFIED.);
#2773=B_SPLINE_CURVE_WITH_KNOTS('',3,(#40607,#40608,#40609,#40610,#40611,
#40612,#40613,#40614,#40615,#40616,#40617,#40618),.UNSPECIFIED.,.F.,.F.,
(4,1,1,1,1,1,1,1,1,4),(65.9734457253856,66.3572419537123,66.8549011483104,
67.3525603429085,67.8502195375065,68.3478787321046,68.8455379267027,69.3431971213007,
69.8408563158988,70.2577934149337),.UNSPECIFIED.);
#2774=B_SPLINE_CURVE_WITH_KNOTS('',3,(#40621,#40622,#40623,#40624,#40625,
#40626,#40627,#40628,#40629,#40630),.UNSPECIFIED.,.F.,.F.,(4,1,1,1,1,1,
1,4),(65.9734457253856,66.0335257266252,66.5311849212233,67.0288441158214,
67.5265033104195,68.0241625050175,68.5218216996156,69.0194808942137),
 .UNSPECIFIED.);
#2775=B_SPLINE_CURVE_WITH_KNOTS('',3,(#40635,#40636,#40637,#40638,#40639,
#40640,#40641,#40642,#40643,#40644,#40645,#40646,#40647,#40648,#40649,#40650,
#40651),.UNSPECIFIED.,.F.,.F.,(4,1,1,1,1,1,1,1,1,1,1,1,1,1,4),(59.690260418206,
59.8876724239374,60.3853316185354,60.8829908131335,61.3806500077316,61.8783092023296,
62.3759683969277,62.8736275915258,63.3712867861239,63.8689459807219,64.36660517532,
64.8642643699181,65.3619235645162,65.8595827591142,65.9734457253856),
 .UNSPECIFIED.);
#2776=B_SPLINE_CURVE_WITH_KNOTS('',3,(#40652,#40653,#40654,#40655,#40656,
#40657,#40658,#40659,#40660,#40661,#40662,#40663,#40664,#40665,#40666,#40667),
 .UNSPECIFIED.,.F.,.F.,(4,1,1,1,1,1,1,1,1,1,1,1,1,4),(59.6902604182061,
60.0616153914484,60.5592745860464,61.0569337806445,61.5545929752426,62.0522521698407,
62.5499113644387,63.0475705590368,63.5452297536349,64.042888948233,64.540548142831,
65.0382073374291,65.5358665320272,65.9734457253856),.UNSPECIFIED.);
#2777=B_SPLINE_CURVE_WITH_KNOTS('',3,(#40672,#40673,#40674,#40675,#40676,
#40677,#40678,#40679,#40680,#40681,#40682,#40683,#40684,#40685,#40686,#40687,
#40688),.UNSPECIFIED.,.F.,.F.,(4,1,1,1,1,1,1,1,1,1,1,1,1,1,4),(53.4070751110265,
53.4181028941624,53.9157620887605,54.4134212833585,54.9110804779566,55.4087396725547,
55.9063988671528,56.4040580617508,56.9017172563489,57.399376450947,57.8970356455451,
58.3946948401431,58.8923540347412,59.3900132293393,59.690260418206),
 .UNSPECIFIED.);
#2778=B_SPLINE_CURVE_WITH_KNOTS('',3,(#40689,#40690,#40691,#40692,#40693,
#40694,#40695,#40696,#40697,#40698,#40699,#40700,#40701,#40702,#40703,#40704,
#40705),.UNSPECIFIED.,.F.,.F.,(4,1,1,1,1,1,1,1,1,1,1,1,1,1,4),(53.4070751110265,
53.5920458616734,54.0897050562715,54.5873642508696,55.0850234454676,55.5826826400657,
56.0803418346638,56.5780010292619,57.0756602238599,57.573319418458,58.0709786130561,
58.5686378076541,59.0662970022522,59.5639561968503,59.6902604182061),
 .UNSPECIFIED.);
#2779=B_SPLINE_CURVE_WITH_KNOTS('',3,(#40710,#40711,#40712,#40713,#40714,
#40715,#40716,#40717,#40718,#40719,#40720,#40721,#40722,#40723,#40724,#40725),
 .UNSPECIFIED.,.F.,.F.,(4,1,1,1,1,1,1,1,1,1,1,1,1,4),(47.1238898038469,
47.4461925589855,47.9438517535836,48.4415109481817,48.9391701427797,49.4368293373778,
49.9344885319759,50.432147726574,50.929806921172,51.4274661157701,51.9251253103682,
52.4227845049663,52.9204436995643,53.4070751110265),.UNSPECIFIED.);
#2780=B_SPLINE_CURVE_WITH_KNOTS('',3,(#40726,#40727,#40728,#40729,#40730,
#40731,#40732,#40733,#40734,#40735,#40736,#40737,#40738,#40739,#40740,#40741),
 .UNSPECIFIED.,.F.,.F.,(4,1,1,1,1,1,1,1,1,1,1,1,1,4),(47.1238898038469,
47.6201355264965,48.1177947210946,48.6154539156927,49.1131131102908,49.6107723048888,
50.1084314994869,50.606090694085,51.103749888683,51.6014090832811,52.0990682778792,
52.5967274724773,53.0943866670753,53.4070751110265),.UNSPECIFIED.);
#2781=B_SPLINE_CURVE_WITH_KNOTS('',3,(#40746,#40747,#40748,#40749,#40750,
#40751,#40752,#40753,#40754,#40755,#40756,#40757,#40758,#40759,#40760,#40761,
#40762),.UNSPECIFIED.,.F.,.F.,(4,1,1,1,1,1,1,1,1,1,1,1,1,1,4),(40.8407044966673,
40.9766230292106,41.4742822238086,41.9719414184067,42.4696006130048,42.9672598076029,
43.4649190022009,43.962578196799,44.4602373913971,44.9578965859952,45.4555557805932,
45.9532149751913,46.4508741697894,46.9485333643874,47.1238898038469),
 .UNSPECIFIED.);
#2782=B_SPLINE_CURVE_WITH_KNOTS('',3,(#40763,#40764,#40765,#40766,#40767,
#40768,#40769,#40770,#40771,#40772,#40773,#40774,#40775,#40776,#40777,#40778,
#40779),.UNSPECIFIED.,.F.,.F.,(4,1,1,1,1,1,1,1,1,1,1,1,1,1,4),(40.8407044966673,
41.1505659967216,41.6482251913197,42.1458843859177,42.6435435805158,43.1412027751139,
43.638861969712,44.13652116431,44.6341803589081,45.1318395535062,45.6294987481042,
46.1271579427023,46.6248171373004,47.1224763318985,47.1238898038469),
 .UNSPECIFIED.);
#2783=B_SPLINE_CURVE_WITH_KNOTS('',3,(#40784,#40785,#40786,#40787,#40788,
#40789,#40790,#40791,#40792,#40793,#40794,#40795,#40796,#40797,#40798,#40799),
 .UNSPECIFIED.,.F.,.F.,(4,1,1,1,1,1,1,1,1,1,1,1,1,4),(34.5575191894877,
35.0047126940337,35.5023718886318,36.0000310832298,36.4976902778279,36.995349472426,
37.4930086670241,37.9906678616221,38.4883270562202,38.9859862508183,39.4836454454163,
39.9813046400144,40.4789638346125,40.8407044966673),.UNSPECIFIED.);
#2784=B_SPLINE_CURVE_WITH_KNOTS('',3,(#40800,#40801,#40802,#40803,#40804,
#40805,#40806,#40807,#40808,#40809,#40810,#40811,#40812,#40813,#40814,#40815,
#40816),.UNSPECIFIED.,.F.,.F.,(4,1,1,1,1,1,1,1,1,1,1,1,1,1,4),(34.5575191894877,
34.6809964669466,35.1786556615447,35.6763148561428,36.1739740507409,36.6716332453389,
37.169292439937,37.6669516345351,38.1646108291331,38.6622700237312,39.1599292183293,
39.6575884129274,40.1552476075254,40.6529068021235,40.8407044966673),
 .UNSPECIFIED.);
#2785=B_SPLINE_CURVE_WITH_KNOTS('',3,(#40821,#40822,#40823,#40824,#40825,
#40826,#40827,#40828,#40829,#40830,#40831,#40832,#40833,#40834,#40835,#40836,
#40837),.UNSPECIFIED.,.F.,.F.,(4,1,1,1,1,1,1,1,1,1,1,1,1,1,4),(28.2743338823081,
28.5351431642587,29.0328023588568,29.5304615534549,30.0281207480529,30.525779942651,
31.0234391372491,31.5210983318472,32.0187575264452,32.5164167210433,33.0140759156414,
33.5117351102395,34.0093943048375,34.5070534994356,34.5575191894877),
 .UNSPECIFIED.);
#2786=B_SPLINE_CURVE_WITH_KNOTS('',3,(#40838,#40839,#40840,#40841,#40842,
#40843,#40844,#40845,#40846,#40847,#40848,#40849,#40850,#40851,#40852,#40853),
 .UNSPECIFIED.,.F.,.F.,(4,1,1,1,1,1,1,1,1,1,1,1,1,4),(28.2743338823081,
28.7090861317698,29.2067453263678,29.7044045209659,30.202063715564,30.699722910162,
31.1973821047601,31.6950412993582,32.1927004939563,32.6903596885543,33.1880188831524,
33.6856780777505,34.1833372723486,34.5575191894877),.UNSPECIFIED.);
#2787=B_SPLINE_CURVE_WITH_KNOTS('',3,(#40858,#40859,#40860,#40861,#40862,
#40863,#40864,#40865,#40866,#40867,#40868,#40869,#40870,#40871,#40872,#40873,
#40874),.UNSPECIFIED.,.F.,.F.,(4,1,1,1,1,1,1,1,1,1,1,1,1,1,4),(21.9911485751285,
22.0655736344838,22.5632328290818,23.0608920236799,23.558551218278,24.0562104128761,
24.5538696074741,25.0515288020722,25.5491879966703,26.0468471912684,26.5445063858664,
27.0421655804645,27.5398247750626,28.0374839696607,28.2743338823081),
 .UNSPECIFIED.);
#2788=B_SPLINE_CURVE_WITH_KNOTS('',3,(#40875,#40876,#40877,#40878,#40879,
#40880,#40881,#40882,#40883,#40884,#40885,#40886,#40887,#40888,#40889,#40890,
#40891),.UNSPECIFIED.,.F.,.F.,(4,1,1,1,1,1,1,1,1,1,1,1,1,1,4),(21.9911485751285,
22.2395166019948,22.7371757965929,23.2348349911909,23.732494185789,24.2301533803871,
24.7278125749852,25.2254717695832,25.7231309641813,26.2207901587794,26.7184493533775,
27.2161085479755,27.7137677425736,28.2114269371717,28.2743338823081),
 .UNSPECIFIED.);
#2789=B_SPLINE_CURVE_WITH_KNOTS('',3,(#40896,#40897,#40898,#40899,#40900,
#40901,#40902,#40903,#40904,#40905,#40906,#40907,#40908,#40909,#40910,#40911),
 .UNSPECIFIED.,.F.,.F.,(4,1,1,1,1,1,1,1,1,1,1,1,1,4),(15.7079632679489,
16.0936632993069,16.591322493905,17.088981688503,17.5866408831011,18.0843000776992,
18.5819592722973,19.0796184668953,19.5772776614934,20.0749368560915,20.5725960506896,
21.0702552452876,21.5679144398857,21.9911485751285),.UNSPECIFIED.);
#2790=B_SPLINE_CURVE_WITH_KNOTS('',3,(#40912,#40913,#40914,#40915,#40916,
#40917,#40918,#40919,#40920,#40921,#40922,#40923,#40924,#40925,#40926,#40927,
#40928),.UNSPECIFIED.,.F.,.F.,(4,1,1,1,1,1,1,1,1,1,1,1,1,1,4),(15.7079632679489,
15.7699470722198,16.2676062668179,16.765265461416,17.2629246560141,17.7605838506121,
18.2582430452102,18.7559022398083,19.2535614344064,19.7512206290044,20.2488798236025,
20.7465390182006,21.2441982127987,21.7418574073967,21.9911485751285),
 .UNSPECIFIED.);
#2791=B_SPLINE_CURVE_WITH_KNOTS('',3,(#41430,#41431,#41432,#41433,#41434,
#41435,#41436,#41437,#41438,#41439,#41440,#41441,#41442,#41443,#41444,#41445,
#41446,#41447,#41448,#41449,#41450,#41451,#41452,#41453,#41454,#41455,#41456,
#41457,#41458,#41459,#41460,#41461,#41462,#41463,#41464,#41465,#41466,#41467,
#41468,#41469,#41470,#41471,#41472,#41473,#41474,#41475,#41476,#41477,#41478,
#41479,#41480,#41481,#41482,#41483,#41484,#41485,#41486,#41487,#41488,#41489,
#41490,#41491,#41492,#41493,#41494,#41495,#41496,#41497,#41498,#41499,#41500,
#41501,#41502,#41503,#41504,#41505,#41506,#41507,#41508,#41509,#41510,#41511,
#41512,#41513,#41514,#41515,#41516,#41517,#41518,#41519,#41520,#41521,#41522,
#41523,#41524,#41525,#41526,#41527,#41528,#41529,#41530,#41531,#41532,#41533,
#41534,#41535,#41536,#41537,#41538,#41539,#41540,#41541,#41542,#41543,#41544,
#41545,#41546,#41547),.UNSPECIFIED.,.F.,.F.,(4,3,3,3,3,3,3,3,3,3,3,3,3,
3,3,3,3,3,3,3,3,3,3,3,3,3,3,3,3,3,3,3,3,3,3,3,3,3,3,4),(0.,0.0640389508670487,
0.126232635496461,0.188657039277152,0.250776918005212,0.301501483646333,
0.311103047329612,0.372484856250651,0.43360723014164,0.453675180569697,
0.515140939082644,0.576285345103759,0.594633063449029,0.605631449437402,
0.61301147768363,0.673473436401074,0.733894290152365,0.793562507830594,
0.833267193557858,0.879431537146101,0.893527612392673,0.900861755744641,
0.959992814090244,1.02064009613363,1.07986501715205,1.14122347970793,1.17190271098587,
1.1856790179708,1.19313842944556,1.2025819422638,1.26115034772533,1.31989387337031,
1.35006824439312,1.3643068112087,1.37388684239216,1.38132579651358,1.43936588678999,
1.49709102825393,1.55390796987554,1.56128884155279),.UNSPECIFIED.);
#2792=B_SPLINE_CURVE_WITH_KNOTS('',3,(#41548,#41549,#41550,#41551,#41552,
#41553,#41554,#41555,#41556,#41557),.UNSPECIFIED.,.F.,.F.,(4,3,3,4),(57.6683865721369,
57.7284665733765,58.2261257679746,58.6430628670095),.UNSPECIFIED.);
#2793=B_SPLINE_CURVE_WITH_KNOTS('',3,(#41559,#41560,#41561,#41562,#41563,
#41564,#41565,#41566,#41567,#41568,#41569,#41570,#41571,#41572,#41573,#41574,
#41575,#41576,#41577,#41578,#41579,#41580,#41581,#41582,#41583,#41584,#41585,
#41586,#41587,#41588,#41589,#41590,#41591,#41592,#41593,#41594,#41595,#41596,
#41597,#41598,#41599,#41600,#41601,#41602,#41603,#41604,#41605,#41606,#41607,
#41608,#41609,#41610,#41611,#41612,#41613,#41614,#41615,#41616,#41617,#41618,
#41619,#41620,#41621,#41622,#41623,#41624,#41625,#41626,#41627,#41628,#41629,
#41630,#41631,#41632,#41633,#41634,#41635,#41636,#41637,#41638,#41639,#41640,
#41641,#41642,#41643,#41644,#41645,#41646,#41647,#41648,#41649,#41650,#41651,
#41652,#41653,#41654,#41655,#41656,#41657,#41658,#41659,#41660,#41661,#41662,
#41663,#41664,#41665,#41666,#41667,#41668,#41669,#41670,#41671,#41672,#41673),
 .UNSPECIFIED.,.F.,.F.,(4,3,3,3,3,3,3,3,3,3,3,3,3,3,3,3,3,3,3,3,3,3,3,3,
3,3,3,3,3,3,3,3,3,3,3,3,3,3,4),(-1.5612888415528,-1.50381997927053,-1.44626607638451,
-1.40841603929727,-1.38397573253337,-1.37502188808332,-1.31651898058331,
-1.25777459806667,-1.2006201888766,-1.18830429954325,-1.18030734756907,
-1.14346577968654,-1.08500221787391,-1.0257955428698,-0.966253568289297,
-0.91777400672482,-0.906613929613625,-0.89902907381174,-0.838953330303881,
-0.778441026219316,-0.77233532203139,-0.712209997853756,-0.651759029464709,
-0.619175485541018,-0.60908817917268,-0.601432360210168,-0.540468743341305,
-0.479070773468726,-0.417730405453208,-0.391090678075187,-0.342204343315789,
-0.320816571858552,-0.310234380897366,-0.301157505671209,-0.239985909763509,
-0.177711909468721,-0.11529068844521,-0.0534506659119964,0.),
 .UNSPECIFIED.);
#2794=B_SPLINE_CURVE_WITH_KNOTS('',3,(#41674,#41675,#41676,#41677,#41678,
#41679,#41680,#41681,#41682,#41683,#41684,#41685,#41686,#41687),
 .UNSPECIFIED.,.F.,.F.,(4,1,1,1,1,1,1,1,1,1,1,4),(10.3764180272042,10.7933551262391,
11.2910143208372,11.7886735154353,12.2863327100333,12.7839919046314,13.2816510992295,
13.7793102938275,14.2769694884256,14.7746286830237,15.2722878776218,15.7079632679489),
 .UNSPECIFIED.);
#2795=B_SPLINE_CURVE_WITH_KNOTS('',3,(#41691,#41692,#41693,#41694,#41695,
#41696,#41697,#41698,#41699,#41700,#41701,#41702),.UNSPECIFIED.,.F.,.F.,
(4,1,1,1,1,1,1,1,1,4),(11.6147305479242,12.1123897425223,12.6100489371204,
13.1077081317185,13.6053673263165,14.1030265209146,14.6006857155127,15.0983449101107,
15.5960041047088,15.7079632679489),.UNSPECIFIED.);
#2796=B_SPLINE_CURVE_WITH_KNOTS('',3,(#42204,#42205,#42206,#42207,#42208,
#42209,#42210,#42211,#42212,#42213,#42214,#42215,#42216,#42217,#42218,#42219,
#42220,#42221,#42222,#42223,#42224,#42225,#42226,#42227,#42228,#42229,#42230,
#42231,#42232,#42233,#42234,#42235,#42236,#42237,#42238,#42239,#42240,#42241,
#42242,#42243,#42244,#42245,#42246,#42247,#42248,#42249,#42250,#42251,#42252,
#42253,#42254,#42255,#42256,#42257,#42258,#42259,#42260,#42261,#42262,#42263,
#42264,#42265,#42266,#42267,#42268,#42269,#42270,#42271,#42272,#42273,#42274,
#42275,#42276,#42277,#42278,#42279,#42280,#42281,#42282,#42283,#42284,#42285,
#42286,#42287,#42288,#42289,#42290,#42291,#42292,#42293,#42294,#42295,#42296,
#42297,#42298,#42299,#42300,#42301,#42302,#42303,#42304,#42305,#42306,#42307,
#42308,#42309,#42310,#42311,#42312,#42313,#42314,#42315,#42316,#42317,#42318,
#42319,#42320,#42321),.UNSPECIFIED.,.F.,.F.,(4,3,3,3,3,3,3,3,3,3,3,3,3,
3,3,3,3,3,3,3,3,3,3,3,3,3,3,3,3,3,3,3,3,3,3,3,3,3,3,4),(0.,0.0573839578688757,
0.114590484122352,0.172466904307786,0.230588407369637,0.277342780760038,
0.283471950450586,0.342148786594638,0.401253301161324,0.417605900931242,
0.476403667266598,0.535433861034147,0.552517961785708,0.561030348077734,
0.568192904833271,0.627729231249355,0.68770609069227,0.747626730537876,
0.787875082072579,0.835383058713792,0.846478499762998,0.853725938073134,
0.86163476712092,0.921384582649023,0.983023160787337,1.04403071219776,1.10598480370002,
1.13696184945115,1.14862783597345,1.15683895023771,1.16793889520228,1.22874774584585,
1.29023148370971,1.32364607620725,1.3501106960563,1.35906742929627,1.42129775631956,
1.48369851743659,1.54568460253334,1.55754822368998),.UNSPECIFIED.);
#2797=B_SPLINE_CURVE_WITH_KNOTS('',3,(#42322,#42323,#42324,#42325,#42326,
#42327,#42328,#42329,#42330,#42331,#42332,#42333,#42334,#42335,#42336,#42337,
#42338,#42339,#42340,#42341,#42342,#42343,#42344,#42345,#42346,#42347,#42348,
#42349,#42350,#42351,#42352,#42353,#42354,#42355,#42356,#42357,#42358,#42359,
#42360,#42361,#42362,#42363,#42364,#42365,#42366,#42367,#42368,#42369,#42370,
#42371,#42372,#42373,#42374,#42375,#42376,#42377,#42378,#42379,#42380,#42381,
#42382,#42383,#42384,#42385,#42386,#42387,#42388,#42389,#42390,#42391,#42392,
#42393,#42394,#42395,#42396,#42397,#42398,#42399,#42400,#42401,#42402,#42403,
#42404,#42405,#42406,#42407,#42408,#42409,#42410,#42411,#42412,#42413,#42414,
#42415,#42416,#42417,#42418,#42419,#42420,#42421,#42422,#42423,#42424,#42425,
#42426,#42427,#42428,#42429,#42430,#42431,#42432,#42433,#42434,#42435,#42436),
 .UNSPECIFIED.,.F.,.F.,(4,3,3,3,3,3,3,3,3,3,3,3,3,3,3,3,3,3,3,3,3,3,3,3,
3,3,3,3,3,3,3,3,3,3,3,3,3,3,4),(-1.55754822368999,-1.49369030775179,-1.4313235190698,
-1.39062308635,-1.36715669998756,-1.35596433121764,-1.34727309230324,-1.2855394700848,
-1.2240883864807,-1.16490422189603,-1.15492087119867,-1.14664991405737,
-1.10572005731137,-1.04502187930064,-0.984006782056958,-0.92320309422318,
-0.874174440126947,-0.855865305758246,-0.848822556599067,-0.787955517218659,
-0.72708847783825,-0.667031022725293,-0.607206878858597,-0.576110200997875,
-0.565145179110016,-0.558975853547965,-0.499936666610499,-0.44095175273352,
-0.382672386577637,-0.358433455972822,-0.313629273976219,-0.294027444352705,
-0.283755524046394,-0.27394190140763,-0.216143666927953,-0.158030747047698,
-0.100247716305122,-0.0435718312192328,0.),.UNSPECIFIED.);
#2798=B_SPLINE_CURVE_WITH_KNOTS('',3,(#42437,#42438,#42439,#42440),
 .UNSPECIFIED.,.F.,.F.,(4,4),(-60.714421740965,-60.641900484641),
 .UNSPECIFIED.);
#3307=LINE('',#39786,#3845);
#3308=LINE('',#39819,#3846);
#3309=LINE('',#39903,#3847);
#3310=LINE('',#39993,#3848);
#3311=LINE('',#40083,#3849);
#3312=LINE('',#40167,#3850);
#3313=LINE('',#40257,#3851);
#3314=LINE('',#40344,#3852);
#3315=LINE('',#40431,#3853);
#3316=LINE('',#40521,#3854);
#3317=LINE('',#40605,#3855);
#3318=LINE('',#40634,#3856);
#3319=LINE('',#40671,#3857);
#3320=LINE('',#40709,#3858);
#3321=LINE('',#40745,#3859);
#3322=LINE('',#40783,#3860);
#3323=LINE('',#40820,#3861);
#3324=LINE('',#40857,#3862);
#3325=LINE('',#40895,#3863);
#3326=LINE('',#42454,#3864);
#3327=LINE('',#42457,#3865);
#3328=LINE('',#42468,#3866);
#3329=LINE('',#42471,#3867);
#3330=LINE('',#42482,#3868);
#3331=LINE('',#42485,#3869);
#3332=LINE('',#42490,#3870);
#3333=LINE('',#42499,#3871);
#3334=LINE('',#42505,#3872);
#3845=VECTOR('',#13128,8.);
#3846=VECTOR('',#13133,8.);
#3847=VECTOR('',#13136,8.);
#3848=VECTOR('',#13139,8.);
#3849=VECTOR('',#13142,8.);
#3850=VECTOR('',#13145,8.);
#3851=VECTOR('',#13148,8.);
#3852=VECTOR('',#13151,8.);
#3853=VECTOR('',#13154,8.);
#3854=VECTOR('',#13157,8.);
#3855=VECTOR('',#13160,7.0685);
#3856=VECTOR('',#13165,7.0685);
#3857=VECTOR('',#13168,7.0685);
#3858=VECTOR('',#13171,7.0685);
#3859=VECTOR('',#13174,7.0685);
#3860=VECTOR('',#13177,7.0685);
#3861=VECTOR('',#13180,7.0685);
#3862=VECTOR('',#13183,7.0685);
#3863=VECTOR('',#13186,7.0685);
#3864=VECTOR('',#13209,7.);
#3865=VECTOR('',#13212,6.);
#3866=VECTOR('',#13227,7.);
#3867=VECTOR('',#13230,6.);
#3868=VECTOR('',#13245,7.);
#3869=VECTOR('',#13248,6.);
#3870=VECTOR('',#13255,6.);
#3871=VECTOR('',#13266,12.);
#3872=VECTOR('',#13275,4.);
#4809=VERTEX_POINT('',#39784);
#4810=VERTEX_POINT('',#39785);
#4811=VERTEX_POINT('',#39787);
#4812=VERTEX_POINT('',#39804);
#4813=VERTEX_POINT('',#39817);
#4814=VERTEX_POINT('',#39818);
#4815=VERTEX_POINT('',#39901);
#4816=VERTEX_POINT('',#39902);
#4817=VERTEX_POINT('',#39991);
#4818=VERTEX_POINT('',#39992);
#4819=VERTEX_POINT('',#40081);
#4820=VERTEX_POINT('',#40082);
#4821=VERTEX_POINT('',#40165);
#4822=VERTEX_POINT('',#40166);
#4823=VERTEX_POINT('',#40255);
#4824=VERTEX_POINT('',#40256);
#4825=VERTEX_POINT('',#40342);
#4826=VERTEX_POINT('',#40343);
#4827=VERTEX_POINT('',#40429);
#4828=VERTEX_POINT('',#40430);
#4829=VERTEX_POINT('',#40519);
#4830=VERTEX_POINT('',#40520);
#4831=VERTEX_POINT('',#40603);
#4832=VERTEX_POINT('',#40604);
#4833=VERTEX_POINT('',#40606);
#4834=VERTEX_POINT('',#40619);
#4835=VERTEX_POINT('',#40632);
#4836=VERTEX_POINT('',#40633);
#4837=VERTEX_POINT('',#40669);
#4838=VERTEX_POINT('',#40670);
#4839=VERTEX_POINT('',#40707);
#4840=VERTEX_POINT('',#40708);
#4841=VERTEX_POINT('',#40743);
#4842=VERTEX_POINT('',#40744);
#4843=VERTEX_POINT('',#40781);
#4844=VERTEX_POINT('',#40782);
#4845=VERTEX_POINT('',#40818);
#4846=VERTEX_POINT('',#40819);
#4847=VERTEX_POINT('',#40855);
#4848=VERTEX_POINT('',#40856);
#4849=VERTEX_POINT('',#40893);
#4850=VERTEX_POINT('',#40894);
#4851=VERTEX_POINT('',#41429);
#4852=VERTEX_POINT('',#41558);
#4853=VERTEX_POINT('',#41689);
#4854=VERTEX_POINT('',#42203);
#4855=VERTEX_POINT('',#42444);
#4856=VERTEX_POINT('',#42446);
#4857=VERTEX_POINT('',#42449);
#4858=VERTEX_POINT('',#42451);
#4859=VERTEX_POINT('',#42456);
#4860=VERTEX_POINT('',#42460);
#4861=VERTEX_POINT('',#42463);
#4862=VERTEX_POINT('',#42465);
#4863=VERTEX_POINT('',#42470);
#4864=VERTEX_POINT('',#42474);
#4865=VERTEX_POINT('',#42477);
#4866=VERTEX_POINT('',#42479);
#4867=VERTEX_POINT('',#42484);
#4868=VERTEX_POINT('',#42488);
#4869=VERTEX_POINT('',#42492);
#4870=VERTEX_POINT('',#42495);
#4871=VERTEX_POINT('',#42498);
#4872=VERTEX_POINT('',#42503);
#6287=EDGE_CURVE('',#4809,#4810,#3307,.T.);
#6288=EDGE_CURVE('',#4809,#4811,#2753,.T.);
#6289=EDGE_CURVE('',#4811,#4812,#1995,.F.);
#6290=EDGE_CURVE('',#4812,#4810,#2754,.T.);
#6291=EDGE_CURVE('',#4813,#4814,#3308,.T.);
#6292=EDGE_CURVE('',#4813,#4809,#2755,.T.);
#6293=EDGE_CURVE('',#4810,#4814,#2756,.T.);
#6294=EDGE_CURVE('',#4815,#4816,#3309,.T.);
#6295=EDGE_CURVE('',#4815,#4813,#2757,.T.);
#6296=EDGE_CURVE('',#4814,#4816,#2758,.T.);
#6297=EDGE_CURVE('',#4817,#4818,#3310,.T.);
#6298=EDGE_CURVE('',#4817,#4815,#2759,.T.);
#6299=EDGE_CURVE('',#4816,#4818,#2760,.T.);
#6300=EDGE_CURVE('',#4819,#4820,#3311,.T.);
#6301=EDGE_CURVE('',#4819,#4817,#2761,.T.);
#6302=EDGE_CURVE('',#4818,#4820,#2762,.T.);
#6303=EDGE_CURVE('',#4821,#4822,#3312,.T.);
#6304=EDGE_CURVE('',#4821,#4819,#2763,.T.);
#6305=EDGE_CURVE('',#4820,#4822,#2764,.T.);
#6306=EDGE_CURVE('',#4823,#4824,#3313,.T.);
#6307=EDGE_CURVE('',#4823,#4821,#2765,.T.);
#6308=EDGE_CURVE('',#4822,#4824,#2766,.T.);
#6309=EDGE_CURVE('',#4825,#4826,#3314,.T.);
#6310=EDGE_CURVE('',#4825,#4823,#2767,.T.);
#6311=EDGE_CURVE('',#4824,#4826,#2768,.T.);
#6312=EDGE_CURVE('',#4827,#4828,#3315,.T.);
#6313=EDGE_CURVE('',#4827,#4825,#2769,.T.);
#6314=EDGE_CURVE('',#4826,#4828,#2770,.T.);
#6315=EDGE_CURVE('',#4829,#4830,#3316,.T.);
#6316=EDGE_CURVE('',#4829,#4827,#2771,.T.);
#6317=EDGE_CURVE('',#4828,#4830,#2772,.T.);
#6318=EDGE_CURVE('',#4831,#4832,#3317,.T.);
#6319=EDGE_CURVE('',#4831,#4833,#2773,.T.);
#6320=EDGE_CURVE('',#4834,#4833,#1996,.T.);
#6321=EDGE_CURVE('',#4832,#4834,#2774,.T.);
#6322=EDGE_CURVE('',#4835,#4836,#3318,.T.);
#6323=EDGE_CURVE('',#4835,#4831,#2775,.T.);
#6324=EDGE_CURVE('',#4836,#4832,#2776,.T.);
#6325=EDGE_CURVE('',#4837,#4838,#3319,.T.);
#6326=EDGE_CURVE('',#4837,#4835,#2777,.T.);
#6327=EDGE_CURVE('',#4838,#4836,#2778,.T.);
#6328=EDGE_CURVE('',#4839,#4840,#3320,.T.);
#6329=EDGE_CURVE('',#4839,#4837,#2779,.T.);
#6330=EDGE_CURVE('',#4840,#4838,#2780,.T.);
#6331=EDGE_CURVE('',#4841,#4842,#3321,.T.);
#6332=EDGE_CURVE('',#4841,#4839,#2781,.T.);
#6333=EDGE_CURVE('',#4842,#4840,#2782,.T.);
#6334=EDGE_CURVE('',#4843,#4844,#3322,.T.);
#6335=EDGE_CURVE('',#4843,#4841,#2783,.T.);
#6336=EDGE_CURVE('',#4844,#4842,#2784,.T.);
#6337=EDGE_CURVE('',#4845,#4846,#3323,.T.);
#6338=EDGE_CURVE('',#4845,#4843,#2785,.T.);
#6339=EDGE_CURVE('',#4846,#4844,#2786,.T.);
#6340=EDGE_CURVE('',#4847,#4848,#3324,.T.);
#6341=EDGE_CURVE('',#4847,#4845,#2787,.T.);
#6342=EDGE_CURVE('',#4848,#4846,#2788,.T.);
#6343=EDGE_CURVE('',#4849,#4850,#3325,.T.);
#6344=EDGE_CURVE('',#4849,#4847,#2789,.T.);
#6345=EDGE_CURVE('',#4850,#4848,#2790,.T.);
#6346=EDGE_CURVE('',#4851,#4834,#2791,.T.);
#6347=EDGE_CURVE('',#4830,#4851,#2792,.T.);
#6348=EDGE_CURVE('',#4852,#4812,#2793,.T.);
#6349=EDGE_CURVE('',#4852,#4850,#2794,.T.);
#6350=EDGE_CURVE('',#4853,#4852,#1997,.T.);
#6351=EDGE_CURVE('',#4853,#4849,#2795,.T.);
#6352=EDGE_CURVE('',#4833,#4854,#2796,.T.);
#6353=EDGE_CURVE('',#4811,#4853,#2797,.T.);
#6354=EDGE_CURVE('',#4854,#4829,#2798,.T.);
#6355=EDGE_CURVE('',#4854,#4851,#1998,.F.);
#6356=EDGE_CURVE('',#4855,#4855,#1999,.T.);
#6357=EDGE_CURVE('',#4856,#4856,#2000,.T.);
#6358=EDGE_CURVE('',#4857,#4857,#2001,.T.);
#6359=EDGE_CURVE('',#4858,#4858,#2002,.T.);
#6360=EDGE_CURVE('',#4855,#4857,#3326,.T.);
#6361=EDGE_CURVE('',#4858,#4859,#3327,.T.);
#6362=EDGE_CURVE('',#4859,#4859,#2003,.T.);
#6363=EDGE_CURVE('',#4860,#4860,#2004,.T.);
#6364=EDGE_CURVE('',#4861,#4861,#2005,.T.);
#6365=EDGE_CURVE('',#4862,#4862,#2006,.T.);
#6366=EDGE_CURVE('',#4860,#4861,#3328,.T.);
#6367=EDGE_CURVE('',#4862,#4863,#3329,.T.);
#6368=EDGE_CURVE('',#4863,#4863,#2007,.T.);
#6369=EDGE_CURVE('',#4864,#4864,#2008,.T.);
#6370=EDGE_CURVE('',#4865,#4865,#2009,.T.);
#6371=EDGE_CURVE('',#4866,#4866,#2010,.T.);
#6372=EDGE_CURVE('',#4864,#4865,#3330,.T.);
#6373=EDGE_CURVE('',#4866,#4867,#3331,.T.);
#6374=EDGE_CURVE('',#4867,#4867,#2011,.T.);
#6375=EDGE_CURVE('',#4868,#4868,#2012,.T.);
#6376=EDGE_CURVE('',#4868,#4856,#3332,.T.);
#6377=EDGE_CURVE('',#4869,#4869,#2013,.T.);
#6378=EDGE_CURVE('',#4870,#4870,#2014,.T.);
#6379=EDGE_CURVE('',#4870,#4871,#3333,.T.);
#6380=EDGE_CURVE('',#4871,#4871,#2015,.T.);
#6381=EDGE_CURVE('',#4872,#4872,#2016,.T.);
#6382=EDGE_CURVE('',#4872,#4869,#3334,.T.);
#9209=ORIENTED_EDGE('',*,*,#6287,.F.);
#9210=ORIENTED_EDGE('',*,*,#6288,.T.);
#9211=ORIENTED_EDGE('',*,*,#6289,.T.);
#9212=ORIENTED_EDGE('',*,*,#6290,.T.);
#9213=ORIENTED_EDGE('',*,*,#6291,.F.);
#9214=ORIENTED_EDGE('',*,*,#6292,.T.);
#9215=ORIENTED_EDGE('',*,*,#6287,.T.);
#9216=ORIENTED_EDGE('',*,*,#6293,.T.);
#9217=ORIENTED_EDGE('',*,*,#6294,.F.);
#9218=ORIENTED_EDGE('',*,*,#6295,.T.);
#9219=ORIENTED_EDGE('',*,*,#6291,.T.);
#9220=ORIENTED_EDGE('',*,*,#6296,.T.);
#9221=ORIENTED_EDGE('',*,*,#6297,.F.);
#9222=ORIENTED_EDGE('',*,*,#6298,.T.);
#9223=ORIENTED_EDGE('',*,*,#6294,.T.);
#9224=ORIENTED_EDGE('',*,*,#6299,.T.);
#9225=ORIENTED_EDGE('',*,*,#6300,.F.);
#9226=ORIENTED_EDGE('',*,*,#6301,.T.);
#9227=ORIENTED_EDGE('',*,*,#6297,.T.);
#9228=ORIENTED_EDGE('',*,*,#6302,.T.);
#9229=ORIENTED_EDGE('',*,*,#6303,.F.);
#9230=ORIENTED_EDGE('',*,*,#6304,.T.);
#9231=ORIENTED_EDGE('',*,*,#6300,.T.);
#9232=ORIENTED_EDGE('',*,*,#6305,.T.);
#9233=ORIENTED_EDGE('',*,*,#6306,.F.);
#9234=ORIENTED_EDGE('',*,*,#6307,.T.);
#9235=ORIENTED_EDGE('',*,*,#6303,.T.);
#9236=ORIENTED_EDGE('',*,*,#6308,.T.);
#9237=ORIENTED_EDGE('',*,*,#6309,.F.);
#9238=ORIENTED_EDGE('',*,*,#6310,.T.);
#9239=ORIENTED_EDGE('',*,*,#6306,.T.);
#9240=ORIENTED_EDGE('',*,*,#6311,.T.);
#9241=ORIENTED_EDGE('',*,*,#6312,.F.);
#9242=ORIENTED_EDGE('',*,*,#6313,.T.);
#9243=ORIENTED_EDGE('',*,*,#6309,.T.);
#9244=ORIENTED_EDGE('',*,*,#6314,.T.);
#9245=ORIENTED_EDGE('',*,*,#6315,.F.);
#9246=ORIENTED_EDGE('',*,*,#6316,.T.);
#9247=ORIENTED_EDGE('',*,*,#6312,.T.);
#9248=ORIENTED_EDGE('',*,*,#6317,.T.);
#9249=ORIENTED_EDGE('',*,*,#6318,.F.);
#9250=ORIENTED_EDGE('',*,*,#6319,.T.);
#9251=ORIENTED_EDGE('',*,*,#6320,.F.);
#9252=ORIENTED_EDGE('',*,*,#6321,.F.);
#9253=ORIENTED_EDGE('',*,*,#6322,.F.);
#9254=ORIENTED_EDGE('',*,*,#6323,.T.);
#9255=ORIENTED_EDGE('',*,*,#6318,.T.);
#9256=ORIENTED_EDGE('',*,*,#6324,.F.);
#9257=ORIENTED_EDGE('',*,*,#6325,.F.);
#9258=ORIENTED_EDGE('',*,*,#6326,.T.);
#9259=ORIENTED_EDGE('',*,*,#6322,.T.);
#9260=ORIENTED_EDGE('',*,*,#6327,.F.);
#9261=ORIENTED_EDGE('',*,*,#6328,.F.);
#9262=ORIENTED_EDGE('',*,*,#6329,.T.);
#9263=ORIENTED_EDGE('',*,*,#6325,.T.);
#9264=ORIENTED_EDGE('',*,*,#6330,.F.);
#9265=ORIENTED_EDGE('',*,*,#6331,.F.);
#9266=ORIENTED_EDGE('',*,*,#6332,.T.);
#9267=ORIENTED_EDGE('',*,*,#6328,.T.);
#9268=ORIENTED_EDGE('',*,*,#6333,.F.);
#9269=ORIENTED_EDGE('',*,*,#6334,.F.);
#9270=ORIENTED_EDGE('',*,*,#6335,.T.);
#9271=ORIENTED_EDGE('',*,*,#6331,.T.);
#9272=ORIENTED_EDGE('',*,*,#6336,.F.);
#9273=ORIENTED_EDGE('',*,*,#6337,.F.);
#9274=ORIENTED_EDGE('',*,*,#6338,.T.);
#9275=ORIENTED_EDGE('',*,*,#6334,.T.);
#9276=ORIENTED_EDGE('',*,*,#6339,.F.);
#9277=ORIENTED_EDGE('',*,*,#6340,.F.);
#9278=ORIENTED_EDGE('',*,*,#6341,.T.);
#9279=ORIENTED_EDGE('',*,*,#6337,.T.);
#9280=ORIENTED_EDGE('',*,*,#6342,.F.);
#9281=ORIENTED_EDGE('',*,*,#6343,.F.);
#9282=ORIENTED_EDGE('',*,*,#6344,.T.);
#9283=ORIENTED_EDGE('',*,*,#6340,.T.);
#9284=ORIENTED_EDGE('',*,*,#6345,.F.);
#9285=ORIENTED_EDGE('',*,*,#6346,.F.);
#9286=ORIENTED_EDGE('',*,*,#6347,.F.);
#9287=ORIENTED_EDGE('',*,*,#6317,.F.);
#9288=ORIENTED_EDGE('',*,*,#6314,.F.);
#9289=ORIENTED_EDGE('',*,*,#6311,.F.);
#9290=ORIENTED_EDGE('',*,*,#6308,.F.);
#9291=ORIENTED_EDGE('',*,*,#6305,.F.);
#9292=ORIENTED_EDGE('',*,*,#6302,.F.);
#9293=ORIENTED_EDGE('',*,*,#6299,.F.);
#9294=ORIENTED_EDGE('',*,*,#6296,.F.);
#9295=ORIENTED_EDGE('',*,*,#6293,.F.);
#9296=ORIENTED_EDGE('',*,*,#6290,.F.);
#9297=ORIENTED_EDGE('',*,*,#6348,.F.);
#9298=ORIENTED_EDGE('',*,*,#6349,.T.);
#9299=ORIENTED_EDGE('',*,*,#6345,.T.);
#9300=ORIENTED_EDGE('',*,*,#6342,.T.);
#9301=ORIENTED_EDGE('',*,*,#6339,.T.);
#9302=ORIENTED_EDGE('',*,*,#6336,.T.);
#9303=ORIENTED_EDGE('',*,*,#6333,.T.);
#9304=ORIENTED_EDGE('',*,*,#6330,.T.);
#9305=ORIENTED_EDGE('',*,*,#6327,.T.);
#9306=ORIENTED_EDGE('',*,*,#6324,.T.);
#9307=ORIENTED_EDGE('',*,*,#6321,.T.);
#9308=ORIENTED_EDGE('',*,*,#6343,.T.);
#9309=ORIENTED_EDGE('',*,*,#6349,.F.);
#9310=ORIENTED_EDGE('',*,*,#6350,.F.);
#9311=ORIENTED_EDGE('',*,*,#6351,.T.);
#9312=ORIENTED_EDGE('',*,*,#6352,.F.);
#9313=ORIENTED_EDGE('',*,*,#6319,.F.);
#9314=ORIENTED_EDGE('',*,*,#6323,.F.);
#9315=ORIENTED_EDGE('',*,*,#6326,.F.);
#9316=ORIENTED_EDGE('',*,*,#6329,.F.);
#9317=ORIENTED_EDGE('',*,*,#6332,.F.);
#9318=ORIENTED_EDGE('',*,*,#6335,.F.);
#9319=ORIENTED_EDGE('',*,*,#6338,.F.);
#9320=ORIENTED_EDGE('',*,*,#6341,.F.);
#9321=ORIENTED_EDGE('',*,*,#6344,.F.);
#9322=ORIENTED_EDGE('',*,*,#6351,.F.);
#9323=ORIENTED_EDGE('',*,*,#6353,.F.);
#9324=ORIENTED_EDGE('',*,*,#6288,.F.);
#9325=ORIENTED_EDGE('',*,*,#6292,.F.);
#9326=ORIENTED_EDGE('',*,*,#6295,.F.);
#9327=ORIENTED_EDGE('',*,*,#6298,.F.);
#9328=ORIENTED_EDGE('',*,*,#6301,.F.);
#9329=ORIENTED_EDGE('',*,*,#6304,.F.);
#9330=ORIENTED_EDGE('',*,*,#6307,.F.);
#9331=ORIENTED_EDGE('',*,*,#6310,.F.);
#9332=ORIENTED_EDGE('',*,*,#6313,.F.);
#9333=ORIENTED_EDGE('',*,*,#6316,.F.);
#9334=ORIENTED_EDGE('',*,*,#6354,.F.);
#9335=ORIENTED_EDGE('',*,*,#6315,.T.);
#9336=ORIENTED_EDGE('',*,*,#6347,.T.);
#9337=ORIENTED_EDGE('',*,*,#6355,.F.);
#9338=ORIENTED_EDGE('',*,*,#6354,.T.);
#9339=ORIENTED_EDGE('',*,*,#6356,.T.);
#9340=ORIENTED_EDGE('',*,*,#6357,.F.);
#9341=ORIENTED_EDGE('',*,*,#6358,.F.);
#9342=ORIENTED_EDGE('',*,*,#6359,.F.);
#9343=ORIENTED_EDGE('',*,*,#6356,.F.);
#9344=ORIENTED_EDGE('',*,*,#6360,.T.);
#9345=ORIENTED_EDGE('',*,*,#6358,.T.);
#9346=ORIENTED_EDGE('',*,*,#6360,.F.);
#9347=ORIENTED_EDGE('',*,*,#6359,.T.);
#9348=ORIENTED_EDGE('',*,*,#6361,.T.);
#9349=ORIENTED_EDGE('',*,*,#6362,.T.);
#9350=ORIENTED_EDGE('',*,*,#6361,.F.);
#9351=ORIENTED_EDGE('',*,*,#6363,.T.);
#9352=ORIENTED_EDGE('',*,*,#6362,.F.);
#9353=ORIENTED_EDGE('',*,*,#6364,.F.);
#9354=ORIENTED_EDGE('',*,*,#6365,.F.);
#9355=ORIENTED_EDGE('',*,*,#6363,.F.);
#9356=ORIENTED_EDGE('',*,*,#6366,.T.);
#9357=ORIENTED_EDGE('',*,*,#6364,.T.);
#9358=ORIENTED_EDGE('',*,*,#6366,.F.);
#9359=ORIENTED_EDGE('',*,*,#6365,.T.);
#9360=ORIENTED_EDGE('',*,*,#6367,.T.);
#9361=ORIENTED_EDGE('',*,*,#6368,.T.);
#9362=ORIENTED_EDGE('',*,*,#6367,.F.);
#9363=ORIENTED_EDGE('',*,*,#6369,.T.);
#9364=ORIENTED_EDGE('',*,*,#6368,.F.);
#9365=ORIENTED_EDGE('',*,*,#6370,.F.);
#9366=ORIENTED_EDGE('',*,*,#6371,.F.);
#9367=ORIENTED_EDGE('',*,*,#6369,.F.);
#9368=ORIENTED_EDGE('',*,*,#6372,.T.);
#9369=ORIENTED_EDGE('',*,*,#6370,.T.);
#9370=ORIENTED_EDGE('',*,*,#6372,.F.);
#9371=ORIENTED_EDGE('',*,*,#6371,.T.);
#9372=ORIENTED_EDGE('',*,*,#6373,.T.);
#9373=ORIENTED_EDGE('',*,*,#6374,.T.);
#9374=ORIENTED_EDGE('',*,*,#6373,.F.);
#9375=ORIENTED_EDGE('',*,*,#6375,.F.);
#9376=ORIENTED_EDGE('',*,*,#6376,.T.);
#9377=ORIENTED_EDGE('',*,*,#6357,.T.);
#9378=ORIENTED_EDGE('',*,*,#6376,.F.);
#9379=ORIENTED_EDGE('',*,*,#6374,.F.);
#9380=ORIENTED_EDGE('',*,*,#6377,.F.);
#9381=ORIENTED_EDGE('',*,*,#6378,.T.);
#9382=ORIENTED_EDGE('',*,*,#6353,.T.);
#9383=ORIENTED_EDGE('',*,*,#6350,.T.);
#9384=ORIENTED_EDGE('',*,*,#6348,.T.);
#9385=ORIENTED_EDGE('',*,*,#6289,.F.);
#9386=ORIENTED_EDGE('',*,*,#6378,.F.);
#9387=ORIENTED_EDGE('',*,*,#6379,.T.);
#9388=ORIENTED_EDGE('',*,*,#6380,.T.);
#9389=ORIENTED_EDGE('',*,*,#6379,.F.);
#9390=ORIENTED_EDGE('',*,*,#6380,.F.);
#9391=ORIENTED_EDGE('',*,*,#6375,.T.);
#9392=ORIENTED_EDGE('',*,*,#6381,.F.);
#9393=ORIENTED_EDGE('',*,*,#6382,.T.);
#9394=ORIENTED_EDGE('',*,*,#6377,.T.);
#9395=ORIENTED_EDGE('',*,*,#6382,.F.);
#9396=ORIENTED_EDGE('',*,*,#6352,.T.);
#9397=ORIENTED_EDGE('',*,*,#6355,.T.);
#9398=ORIENTED_EDGE('',*,*,#6346,.T.);
#9399=ORIENTED_EDGE('',*,*,#6320,.T.);
#9400=ORIENTED_EDGE('',*,*,#6381,.T.);
#9807=CYLINDRICAL_SURFACE('',#11160,7.925);
#9808=CYLINDRICAL_SURFACE('',#11162,7.925);
#9809=CYLINDRICAL_SURFACE('',#11163,7.925);
#9810=CYLINDRICAL_SURFACE('',#11164,7.925);
#9811=CYLINDRICAL_SURFACE('',#11165,7.925);
#9812=CYLINDRICAL_SURFACE('',#11166,7.925);
#9813=CYLINDRICAL_SURFACE('',#11167,7.925);
#9814=CYLINDRICAL_SURFACE('',#11168,7.925);
#9815=CYLINDRICAL_SURFACE('',#11169,7.925);
#9816=CYLINDRICAL_SURFACE('',#11170,7.925);
#9817=CYLINDRICAL_SURFACE('',#11171,7.0685);
#9818=CYLINDRICAL_SURFACE('',#11173,7.0685);
#9819=CYLINDRICAL_SURFACE('',#11174,7.0685);
#9820=CYLINDRICAL_SURFACE('',#11175,7.0685);
#9821=CYLINDRICAL_SURFACE('',#11176,7.0685);
#9822=CYLINDRICAL_SURFACE('',#11177,7.0685);
#9823=CYLINDRICAL_SURFACE('',#11178,7.0685);
#9824=CYLINDRICAL_SURFACE('',#11179,7.0685);
#9825=CYLINDRICAL_SURFACE('',#11180,7.0685);
#9826=CYLINDRICAL_SURFACE('',#11181,7.0685);
#9827=CYLINDRICAL_SURFACE('',#11183,7.925);
#9828=CYLINDRICAL_SURFACE('',#11191,7.);
#9829=CYLINDRICAL_SURFACE('',#11192,6.);
#9830=CYLINDRICAL_SURFACE('',#11199,7.);
#9831=CYLINDRICAL_SURFACE('',#11200,6.);
#9832=CYLINDRICAL_SURFACE('',#11207,7.);
#9833=CYLINDRICAL_SURFACE('',#11208,6.);
#9834=CYLINDRICAL_SURFACE('',#11210,6.);
#9835=CYLINDRICAL_SURFACE('',#11216,12.);
#9836=CYLINDRICAL_SURFACE('',#11219,4.);
#10337=ADVANCED_FACE('',(#1101),#9807,.T.);
#10338=ADVANCED_FACE('',(#1102),#9808,.T.);
#10339=ADVANCED_FACE('',(#1103),#9809,.T.);
#10340=ADVANCED_FACE('',(#1104),#9810,.T.);
#10341=ADVANCED_FACE('',(#1105),#9811,.T.);
#10342=ADVANCED_FACE('',(#1106),#9812,.T.);
#10343=ADVANCED_FACE('',(#1107),#9813,.T.);
#10344=ADVANCED_FACE('',(#1108),#9814,.T.);
#10345=ADVANCED_FACE('',(#1109),#9815,.T.);
#10346=ADVANCED_FACE('',(#1110),#9816,.T.);
#10347=ADVANCED_FACE('',(#1111),#9817,.T.);
#10348=ADVANCED_FACE('',(#1112),#9818,.T.);
#10349=ADVANCED_FACE('',(#1113),#9819,.T.);
#10350=ADVANCED_FACE('',(#1114),#9820,.T.);
#10351=ADVANCED_FACE('',(#1115),#9821,.T.);
#10352=ADVANCED_FACE('',(#1116),#9822,.T.);
#10353=ADVANCED_FACE('',(#1117),#9823,.T.);
#10354=ADVANCED_FACE('',(#1118),#9824,.T.);
#10355=ADVANCED_FACE('',(#1119),#9825,.T.);
#10356=ADVANCED_FACE('',(#1120),#601,.F.);
#10357=ADVANCED_FACE('',(#1121),#9826,.T.);
#10358=ADVANCED_FACE('',(#1122),#602,.F.);
#10359=ADVANCED_FACE('',(#1123),#9827,.T.);
#10360=ADVANCED_FACE('',(#1124,#475),#567,.T.);
#10361=ADVANCED_FACE('',(#1125,#476),#568,.F.);
#10362=ADVANCED_FACE('',(#1126),#9828,.T.);
#10363=ADVANCED_FACE('',(#1127),#9829,.T.);
#10364=ADVANCED_FACE('',(#1128,#477),#569,.T.);
#10365=ADVANCED_FACE('',(#1129,#478),#570,.F.);
#10366=ADVANCED_FACE('',(#1130),#9830,.T.);
#10367=ADVANCED_FACE('',(#1131),#9831,.T.);
#10368=ADVANCED_FACE('',(#1132,#479),#571,.T.);
#10369=ADVANCED_FACE('',(#1133,#480),#572,.F.);
#10370=ADVANCED_FACE('',(#1134),#9832,.T.);
#10371=ADVANCED_FACE('',(#1135),#9833,.T.);
#10372=ADVANCED_FACE('',(#1136),#9834,.T.);
#10373=ADVANCED_FACE('',(#1137,#481),#573,.F.);
#10374=ADVANCED_FACE('',(#1138,#482),#574,.T.);
#10375=ADVANCED_FACE('',(#1139),#9835,.T.);
#10376=ADVANCED_FACE('',(#1140,#483),#575,.F.);
#10377=ADVANCED_FACE('',(#1141),#9836,.F.);
#10378=ADVANCED_FACE('',(#1142,#484),#576,.T.);
#10391=CLOSED_SHELL('',(#10337,#10338,#10339,#10340,#10341,#10342,#10343,
#10344,#10345,#10346,#10347,#10348,#10349,#10350,#10351,#10352,#10353,#10354,
#10355,#10356,#10357,#10358,#10359,#10360,#10361,#10362,#10363,#10364,#10365,
#10366,#10367,#10368,#10369,#10370,#10371,#10372,#10373,#10374,#10375,#10376,
#10377,#10378));
#11159=AXIS2_PLACEMENT_3D('',#39782,#13124,#13125);
#11160=AXIS2_PLACEMENT_3D('',#39783,#13126,#13127);
#11161=AXIS2_PLACEMENT_3D('',#39805,#13129,#13130);
#11162=AXIS2_PLACEMENT_3D('',#39816,#13131,#13132);
#11163=AXIS2_PLACEMENT_3D('',#39900,#13134,#13135);
#11164=AXIS2_PLACEMENT_3D('',#39990,#13137,#13138);
#11165=AXIS2_PLACEMENT_3D('',#40080,#13140,#13141);
#11166=AXIS2_PLACEMENT_3D('',#40164,#13143,#13144);
#11167=AXIS2_PLACEMENT_3D('',#40254,#13146,#13147);
#11168=AXIS2_PLACEMENT_3D('',#40341,#13149,#13150);
#11169=AXIS2_PLACEMENT_3D('',#40428,#13152,#13153);
#11170=AXIS2_PLACEMENT_3D('',#40518,#13155,#13156);
#11171=AXIS2_PLACEMENT_3D('',#40602,#13158,#13159);
#11172=AXIS2_PLACEMENT_3D('',#40620,#13161,#13162);
#11173=AXIS2_PLACEMENT_3D('',#40631,#13163,#13164);
#11174=AXIS2_PLACEMENT_3D('',#40668,#13166,#13167);
#11175=AXIS2_PLACEMENT_3D('',#40706,#13169,#13170);
#11176=AXIS2_PLACEMENT_3D('',#40742,#13172,#13173);
#11177=AXIS2_PLACEMENT_3D('',#40780,#13175,#13176);
#11178=AXIS2_PLACEMENT_3D('',#40817,#13178,#13179);
#11179=AXIS2_PLACEMENT_3D('',#40854,#13181,#13182);
#11180=AXIS2_PLACEMENT_3D('',#40892,#13184,#13185);
#11181=AXIS2_PLACEMENT_3D('',#41688,#13187,#13188);
#11182=AXIS2_PLACEMENT_3D('',#41690,#13189,#13190);
#11183=AXIS2_PLACEMENT_3D('',#42441,#13191,#13192);
#11184=AXIS2_PLACEMENT_3D('',#42442,#13193,#13194);
#11185=AXIS2_PLACEMENT_3D('',#42443,#13195,#13196);
#11186=AXIS2_PLACEMENT_3D('',#42445,#13197,#13198);
#11187=AXIS2_PLACEMENT_3D('',#42447,#13199,#13200);
#11188=AXIS2_PLACEMENT_3D('',#42448,#13201,#13202);
#11189=AXIS2_PLACEMENT_3D('',#42450,#13203,#13204);
#11190=AXIS2_PLACEMENT_3D('',#42452,#13205,#13206);
#11191=AXIS2_PLACEMENT_3D('',#42453,#13207,#13208);
#11192=AXIS2_PLACEMENT_3D('',#42455,#13210,#13211);
#11193=AXIS2_PLACEMENT_3D('',#42458,#13213,#13214);
#11194=AXIS2_PLACEMENT_3D('',#42459,#13215,#13216);
#11195=AXIS2_PLACEMENT_3D('',#42461,#13217,#13218);
#11196=AXIS2_PLACEMENT_3D('',#42462,#13219,#13220);
#11197=AXIS2_PLACEMENT_3D('',#42464,#13221,#13222);
#11198=AXIS2_PLACEMENT_3D('',#42466,#13223,#13224);
#11199=AXIS2_PLACEMENT_3D('',#42467,#13225,#13226);
#11200=AXIS2_PLACEMENT_3D('',#42469,#13228,#13229);
#11201=AXIS2_PLACEMENT_3D('',#42472,#13231,#13232);
#11202=AXIS2_PLACEMENT_3D('',#42473,#13233,#13234);
#11203=AXIS2_PLACEMENT_3D('',#42475,#13235,#13236);
#11204=AXIS2_PLACEMENT_3D('',#42476,#13237,#13238);
#11205=AXIS2_PLACEMENT_3D('',#42478,#13239,#13240);
#11206=AXIS2_PLACEMENT_3D('',#42480,#13241,#13242);
#11207=AXIS2_PLACEMENT_3D('',#42481,#13243,#13244);
#11208=AXIS2_PLACEMENT_3D('',#42483,#13246,#13247);
#11209=AXIS2_PLACEMENT_3D('',#42486,#13249,#13250);
#11210=AXIS2_PLACEMENT_3D('',#42487,#13251,#13252);
#11211=AXIS2_PLACEMENT_3D('',#42489,#13253,#13254);
#11212=AXIS2_PLACEMENT_3D('',#42491,#13256,#13257);
#11213=AXIS2_PLACEMENT_3D('',#42493,#13258,#13259);
#11214=AXIS2_PLACEMENT_3D('',#42494,#13260,#13261);
#11215=AXIS2_PLACEMENT_3D('',#42496,#13262,#13263);
#11216=AXIS2_PLACEMENT_3D('',#42497,#13264,#13265);
#11217=AXIS2_PLACEMENT_3D('',#42500,#13267,#13268);
#11218=AXIS2_PLACEMENT_3D('',#42501,#13269,#13270);
#11219=AXIS2_PLACEMENT_3D('',#42502,#13271,#13272);
#11220=AXIS2_PLACEMENT_3D('',#42504,#13273,#13274);
#11221=AXIS2_PLACEMENT_3D('',#42506,#13276,#13277);
#13124=DIRECTION('axis',(0.,0.,1.));
#13125=DIRECTION('refdir',(1.,0.,0.));
#13126=DIRECTION('center_axis',(0.,0.,1.));
#13127=DIRECTION('ref_axis',(1.,0.,0.));
#13128=DIRECTION('',(0.,0.,-1.));
#13129=DIRECTION('center_axis',(0.,0.,-1.));
#13130=DIRECTION('ref_axis',(1.,0.,0.));
#13131=DIRECTION('center_axis',(0.,0.,1.));
#13132=DIRECTION('ref_axis',(1.,0.,0.));
#13133=DIRECTION('',(0.,0.,-1.));
#13134=DIRECTION('center_axis',(0.,0.,1.));
#13135=DIRECTION('ref_axis',(1.,0.,0.));
#13136=DIRECTION('',(0.,0.,-1.));
#13137=DIRECTION('center_axis',(0.,0.,1.));
#13138=DIRECTION('ref_axis',(1.,0.,0.));
#13139=DIRECTION('',(0.,0.,-1.));
#13140=DIRECTION('center_axis',(0.,0.,1.));
#13141=DIRECTION('ref_axis',(1.,0.,0.));
#13142=DIRECTION('',(0.,0.,-1.));
#13143=DIRECTION('center_axis',(0.,0.,1.));
#13144=DIRECTION('ref_axis',(1.,0.,0.));
#13145=DIRECTION('',(0.,0.,-1.));
#13146=DIRECTION('center_axis',(0.,0.,1.));
#13147=DIRECTION('ref_axis',(1.,0.,0.));
#13148=DIRECTION('',(0.,0.,-1.));
#13149=DIRECTION('center_axis',(0.,0.,1.));
#13150=DIRECTION('ref_axis',(1.,0.,0.));
#13151=DIRECTION('',(0.,0.,-1.));
#13152=DIRECTION('center_axis',(0.,0.,1.));
#13153=DIRECTION('ref_axis',(1.,0.,0.));
#13154=DIRECTION('',(0.,0.,-1.));
#13155=DIRECTION('center_axis',(0.,0.,1.));
#13156=DIRECTION('ref_axis',(1.,0.,0.));
#13157=DIRECTION('',(0.,0.,-1.));
#13158=DIRECTION('center_axis',(0.,0.,1.));
#13159=DIRECTION('ref_axis',(0.540789512512072,-0.84115795375004,0.));
#13160=DIRECTION('',(0.,0.,1.));
#13161=DIRECTION('center_axis',(0.,0.,1.));
#13162=DIRECTION('ref_axis',(1.,5.20562201223838E-14,0.));
#13163=DIRECTION('center_axis',(0.,0.,1.));
#13164=DIRECTION('ref_axis',(1.,5.20562201223838E-14,0.));
#13165=DIRECTION('',(0.,0.,1.));
#13166=DIRECTION('center_axis',(0.,0.,1.));
#13167=DIRECTION('ref_axis',(1.,5.20562201223838E-14,0.));
#13168=DIRECTION('',(0.,0.,1.));
#13169=DIRECTION('center_axis',(0.,0.,1.));
#13170=DIRECTION('ref_axis',(1.,5.20562201223838E-14,0.));
#13171=DIRECTION('',(0.,0.,1.));
#13172=DIRECTION('center_axis',(0.,0.,1.));
#13173=DIRECTION('ref_axis',(1.,5.20562201223838E-14,0.));
#13174=DIRECTION('',(0.,0.,1.));
#13175=DIRECTION('center_axis',(0.,0.,1.));
#13176=DIRECTION('ref_axis',(1.,5.20562201223838E-14,0.));
#13177=DIRECTION('',(0.,0.,1.));
#13178=DIRECTION('center_axis',(0.,0.,1.));
#13179=DIRECTION('ref_axis',(1.,5.20562201223838E-14,0.));
#13180=DIRECTION('',(0.,0.,1.));
#13181=DIRECTION('center_axis',(0.,0.,1.));
#13182=DIRECTION('ref_axis',(1.,5.20562201223838E-14,0.));
#13183=DIRECTION('',(0.,0.,1.));
#13184=DIRECTION('center_axis',(0.,0.,1.));
#13185=DIRECTION('ref_axis',(1.,5.20562201223838E-14,0.));
#13186=DIRECTION('',(0.,0.,1.));
#13187=DIRECTION('center_axis',(0.,0.,1.));
#13188=DIRECTION('ref_axis',(0.888917950975616,0.4580664541672,0.));
#13189=DIRECTION('center_axis',(0.,0.,-1.));
#13190=DIRECTION('ref_axis',(1.,5.20562201223838E-14,0.));
#13191=DIRECTION('center_axis',(0.,0.,1.));
#13192=DIRECTION('ref_axis',(1.,0.,0.));
#13193=DIRECTION('center_axis',(0.,0.,-1.));
#13194=DIRECTION('ref_axis',(1.,0.,0.));
#13195=DIRECTION('center_axis',(0.,0.,1.));
#13196=DIRECTION('ref_axis',(1.,0.,0.));
#13197=DIRECTION('center_axis',(0.,0.,1.));
#13198=DIRECTION('ref_axis',(1.,0.,0.));
#13199=DIRECTION('center_axis',(0.,0.,1.));
#13200=DIRECTION('ref_axis',(1.,0.,0.));
#13201=DIRECTION('center_axis',(0.,0.,1.));
#13202=DIRECTION('ref_axis',(1.,0.,0.));
#13203=DIRECTION('center_axis',(0.,0.,1.));
#13204=DIRECTION('ref_axis',(1.,0.,0.));
#13205=DIRECTION('center_axis',(0.,0.,-1.));
#13206=DIRECTION('ref_axis',(1.,0.,0.));
#13207=DIRECTION('center_axis',(0.,0.,1.));
#13208=DIRECTION('ref_axis',(1.,0.,0.));
#13209=DIRECTION('',(0.,0.,-1.));
#13210=DIRECTION('center_axis',(0.,0.,1.));
#13211=DIRECTION('ref_axis',(1.,0.,0.));
#13212=DIRECTION('',(0.,0.,-1.));
#13213=DIRECTION('center_axis',(0.,0.,1.));
#13214=DIRECTION('ref_axis',(1.,0.,0.));
#13215=DIRECTION('center_axis',(0.,0.,1.));
#13216=DIRECTION('ref_axis',(1.,0.,0.));
#13217=DIRECTION('center_axis',(0.,0.,1.));
#13218=DIRECTION('ref_axis',(1.,0.,0.));
#13219=DIRECTION('center_axis',(0.,0.,1.));
#13220=DIRECTION('ref_axis',(1.,0.,0.));
#13221=DIRECTION('center_axis',(0.,0.,1.));
#13222=DIRECTION('ref_axis',(1.,0.,0.));
#13223=DIRECTION('center_axis',(0.,0.,-1.));
#13224=DIRECTION('ref_axis',(1.,0.,0.));
#13225=DIRECTION('center_axis',(0.,0.,1.));
#13226=DIRECTION('ref_axis',(1.,0.,0.));
#13227=DIRECTION('',(0.,0.,-1.));
#13228=DIRECTION('center_axis',(0.,0.,1.));
#13229=DIRECTION('ref_axis',(1.,0.,0.));
#13230=DIRECTION('',(0.,0.,-1.));
#13231=DIRECTION('center_axis',(0.,0.,1.));
#13232=DIRECTION('ref_axis',(1.,0.,0.));
#13233=DIRECTION('center_axis',(0.,0.,1.));
#13234=DIRECTION('ref_axis',(1.,0.,0.));
#13235=DIRECTION('center_axis',(0.,0.,1.));
#13236=DIRECTION('ref_axis',(1.,0.,0.));
#13237=DIRECTION('center_axis',(0.,0.,1.));
#13238=DIRECTION('ref_axis',(1.,0.,0.));
#13239=DIRECTION('center_axis',(0.,0.,1.));
#13240=DIRECTION('ref_axis',(1.,0.,0.));
#13241=DIRECTION('center_axis',(0.,0.,-1.));
#13242=DIRECTION('ref_axis',(1.,0.,0.));
#13243=DIRECTION('center_axis',(0.,0.,1.));
#13244=DIRECTION('ref_axis',(1.,0.,0.));
#13245=DIRECTION('',(0.,0.,-1.));
#13246=DIRECTION('center_axis',(0.,0.,1.));
#13247=DIRECTION('ref_axis',(1.,0.,0.));
#13248=DIRECTION('',(0.,0.,-1.));
#13249=DIRECTION('center_axis',(0.,0.,1.));
#13250=DIRECTION('ref_axis',(1.,0.,0.));
#13251=DIRECTION('center_axis',(0.,0.,1.));
#13252=DIRECTION('ref_axis',(1.,0.,0.));
#13253=DIRECTION('center_axis',(0.,0.,1.));
#13254=DIRECTION('ref_axis',(1.,0.,0.));
#13255=DIRECTION('',(0.,0.,-1.));
#13256=DIRECTION('center_axis',(0.,0.,1.));
#13257=DIRECTION('ref_axis',(1.,0.,0.));
#13258=DIRECTION('center_axis',(0.,0.,-1.));
#13259=DIRECTION('ref_axis',(1.,0.,0.));
#13260=DIRECTION('center_axis',(0.,0.,1.));
#13261=DIRECTION('ref_axis',(1.,0.,0.));
#13262=DIRECTION('center_axis',(0.,0.,1.));
#13263=DIRECTION('ref_axis',(1.,0.,0.));
#13264=DIRECTION('center_axis',(0.,0.,1.));
#13265=DIRECTION('ref_axis',(1.,0.,0.));
#13266=DIRECTION('',(0.,0.,-1.));
#13267=DIRECTION('center_axis',(0.,0.,1.));
#13268=DIRECTION('ref_axis',(1.,0.,0.));
#13269=DIRECTION('center_axis',(0.,0.,1.));
#13270=DIRECTION('ref_axis',(1.,0.,0.));
#13271=DIRECTION('center_axis',(0.,0.,1.));
#13272=DIRECTION('ref_axis',(1.,0.,0.));
#13273=DIRECTION('center_axis',(0.,0.,-1.));
#13274=DIRECTION('ref_axis',(1.,0.,0.));
#13275=DIRECTION('',(0.,0.,-1.));
#13276=DIRECTION('center_axis',(0.,0.,1.));
#13277=DIRECTION('ref_axis',(1.,0.,0.));
#39782=CARTESIAN_POINT('',(0.,0.,0.));
#39783=CARTESIAN_POINT('Origin',(0.,0.,0.));
#39784=CARTESIAN_POINT('',(-7.92502372531584,0.000203888857960161,0.482686825365204));
#39785=CARTESIAN_POINT('',(-7.92493078473506,0.000130763509288048,0.267313174634791));
#39786=CARTESIAN_POINT('',(-7.925,-9.70532588324277E-16,0.));
#39787=CARTESIAN_POINT('',(3.45478907940189,7.13232482552817,0.));
#39788=CARTESIAN_POINT('Ctrl Pts',(-7.92502372531584,0.000203888857960161,
0.482686825365204));
#39789=CARTESIAN_POINT('Ctrl Pts',(-7.92532623227895,0.295954310302644,
0.473777398238157));
#39790=CARTESIAN_POINT('Ctrl Pts',(-7.90908776172729,0.591671595388266,
0.46486797111111));
#39791=CARTESIAN_POINT('Ctrl Pts',(-7.87605276584388,0.88550030186303,0.455958543984063));
#39792=CARTESIAN_POINT('Ctrl Pts',(-7.72921199846845,2.19157077597367,0.416356083586355));
#39793=CARTESIAN_POINT('Ctrl Pts',(-7.25050411141088,3.46032655960519,0.376753623188647));
#39794=CARTESIAN_POINT('Ctrl Pts',(-6.49799558141544,4.53787932192357,0.33715116279094));
#39795=CARTESIAN_POINT('Ctrl Pts',(-5.74548705142,5.61543208424195,0.297548702393232));
#39796=CARTESIAN_POINT('Ctrl Pts',(-4.7191778784867,6.50178182524719,0.257946241995526));
#39797=CARTESIAN_POINT('Ctrl Pts',(-3.54355620222258,7.0893994069169,0.218343781597818));
#39798=CARTESIAN_POINT('Ctrl Pts',(-2.36793452595845,7.67701698858661,0.178741321200111));
#39799=CARTESIAN_POINT('Ctrl Pts',(-1.04300034636349,7.96590241092079,0.139138860802403));
#39800=CARTESIAN_POINT('Ctrl Pts',(0.270533623218387,7.92104793571692,0.0995364004046956));
#39801=CARTESIAN_POINT('Ctrl Pts',(1.37100770006842,7.88346901630132,0.0663576002697969));
#39802=CARTESIAN_POINT('Ctrl Pts',(2.46347993683329,7.61163710618861,0.0331788001348983));
#39803=CARTESIAN_POINT('Ctrl Pts',(3.45507168555157,7.13251860299055,-2.84060969191202E-16));
#39804=CARTESIAN_POINT('',(-3.45478907940191,7.13232482552816,0.));
#39805=CARTESIAN_POINT('Origin',(0.,0.,0.));
#39806=CARTESIAN_POINT('Ctrl Pts',(-3.45478907940191,7.13232482552816,6.24500451351651E-16));
#39807=CARTESIAN_POINT('Ctrl Pts',(-4.63794475549662,6.55922230860771,0.0396024603977076));
#39808=CARTESIAN_POINT('Ctrl Pts',(-5.67516414283391,5.6863469211646,0.0792049207954145));
#39809=CARTESIAN_POINT('Ctrl Pts',(-6.44101552295666,4.61843342960788,0.118807381193121));
#39810=CARTESIAN_POINT('Ctrl Pts',(-7.20686690307942,3.55051993805114,0.158409841590829));
#39811=CARTESIAN_POINT('Ctrl Pts',(-7.70135027598763,2.28756834238077,0.198012301988537));
#39812=CARTESIAN_POINT('Ctrl Pts',(-7.86443494073275,0.983361388757709,
0.237614762386245));
#39813=CARTESIAN_POINT('Ctrl Pts',(-7.90520139443602,0.657347336624382,
0.24751423313576));
#39814=CARTESIAN_POINT('Ctrl Pts',(-7.92526021663928,0.328755420640525,
0.257413703885276));
#39815=CARTESIAN_POINT('Ctrl Pts',(-7.92493078473506,0.000130763509288048,
0.267313174634791));
#39816=CARTESIAN_POINT('Origin',(0.,0.,0.));
#39817=CARTESIAN_POINT('',(-7.92532948546385,-0.000170658577658411,1.9826868253652));
#39818=CARTESIAN_POINT('',(-7.92542130335282,-0.000150527452605021,1.76731317463479));
#39819=CARTESIAN_POINT('',(-7.925,-9.70532588324277E-16,0.));
#39820=CARTESIAN_POINT('Ctrl Pts',(-7.92532948546385,-0.000170658577658411,
1.9826868253652));
#39821=CARTESIAN_POINT('Ctrl Pts',(-7.92427024157546,1.11771666749154,1.94900692301065));
#39822=CARTESIAN_POINT('Ctrl Pts',(-7.68542693347382,2.23604223578417,1.91532702065609));
#39823=CARTESIAN_POINT('Ctrl Pts',(-7.22635584668683,3.25516459727708,1.88164711830153));
#39824=CARTESIAN_POINT('Ctrl Pts',(-6.68655782878211,4.45349802878656,1.84204465790382));
#39825=CARTESIAN_POINT('Ctrl Pts',(-5.84226858153731,5.5146711684689,1.80244219750611));
#39826=CARTESIAN_POINT('Ctrl Pts',(-4.7958983657642,6.30996626240027,1.76283973710841));
#39827=CARTESIAN_POINT('Ctrl Pts',(-3.7495281499911,7.10526135633162,1.7232372767107));
#39828=CARTESIAN_POINT('Ctrl Pts',(-2.50107696568969,7.634678404512,1.68363481631299));
#39829=CARTESIAN_POINT('Ctrl Pts',(-1.20197894693782,7.83400038341452,1.64403235591528));
#39830=CARTESIAN_POINT('Ctrl Pts',(0.0971190718140523,8.03332236231703,
1.60442989551758));
#39831=CARTESIAN_POINT('Ctrl Pts',(1.4468639250164,7.90254927194168,1.56482743511987));
#39832=CARTESIAN_POINT('Ctrl Pts',(2.68353479884886,7.4575435850056,1.52522497472216));
#39833=CARTESIAN_POINT('Ctrl Pts',(3.92020567268132,7.01253789806953,1.48562251432445));
#39834=CARTESIAN_POINT('Ctrl Pts',(5.04380256714389,6.25329961457273,1.44602005392675));
#39835=CARTESIAN_POINT('Ctrl Pts',(5.91803587468444,5.27192249672745,1.40641759352904));
#39836=CARTESIAN_POINT('Ctrl Pts',(6.79226918222501,4.29054537888217,1.36681513313133));
#39837=CARTESIAN_POINT('Ctrl Pts',(7.41713890284356,3.08702942668839,1.32721267273363));
#39838=CARTESIAN_POINT('Ctrl Pts',(7.71684983649437,1.8073582788516,1.28761021233592));
#39839=CARTESIAN_POINT('Ctrl Pts',(8.01656077014517,0.527687131014814,1.24800775193821));
#39840=CARTESIAN_POINT('Ctrl Pts',(7.99111291682824,-0.828139212464995,
1.2084052915405));
#39841=CARTESIAN_POINT('Ctrl Pts',(7.64359304336192,-2.09566234689561,1.1688028311428));
#39842=CARTESIAN_POINT('Ctrl Pts',(7.29607316989561,-3.36318548132621,1.12920037074509));
#39843=CARTESIAN_POINT('Ctrl Pts',(6.62648127627991,-4.54240540670763,1.08959791034738));
#39844=CARTESIAN_POINT('Ctrl Pts',(5.71603724686592,-5.49028541995301,1.04999544994967));
#39845=CARTESIAN_POINT('Ctrl Pts',(4.80559321745193,-6.4381654331984,1.01039298955197));
#39846=CARTESIAN_POINT('Ctrl Pts',(3.65429705223965,-7.15470553430775,0.970790529154259));
#39847=CARTESIAN_POINT('Ctrl Pts',(2.40179822718111,-7.55299143001374,0.931188068756552));
#39848=CARTESIAN_POINT('Ctrl Pts',(1.14929940212257,-7.95127732571973,0.891585608358844));
#39849=CARTESIAN_POINT('Ctrl Pts',(-0.204402082782219,-8.03130901602234,
0.851983147961137));
#39850=CARTESIAN_POINT('Ctrl Pts',(-1.49510550858021,-7.78337825673035,
0.81238068756343));
#39851=CARTESIAN_POINT('Ctrl Pts',(-2.78580893437819,-7.53544749743836,
0.772778227165722));
#39852=CARTESIAN_POINT('Ctrl Pts',(-4.01351430106938,-6.95955428855176,
0.733175766768014));
#39853=CARTESIAN_POINT('Ctrl Pts',(-5.02930384455586,-6.12555425440213,
0.693573306370307));
#39854=CARTESIAN_POINT('Ctrl Pts',(-6.04509338804233,-5.29155422025249,
0.6539708459726));
#39855=CARTESIAN_POINT('Ctrl Pts',(-6.84896710832411,-4.19944736083982,
0.614368385574893));
#39856=CARTESIAN_POINT('Ctrl Pts',(-7.34341714461835,-2.98170134883861,
0.574765925177185));
#39857=CARTESIAN_POINT('Ctrl Pts',(-7.72662998700875,-2.03791355166095,
0.544072891906525));
#39858=CARTESIAN_POINT('Ctrl Pts',(-7.92398158689877,-1.01865819910462,
0.513379858635864));
#39859=CARTESIAN_POINT('Ctrl Pts',(-7.92502372531584,0.000203888857960161,
0.482686825365204));
#39860=CARTESIAN_POINT('Ctrl Pts',(-7.92493078473506,0.000130763509288048,
0.267313174634791));
#39861=CARTESIAN_POINT('Ctrl Pts',(-7.92394233669697,-0.985895160087429,
0.297016164282983));
#39862=CARTESIAN_POINT('Ctrl Pts',(-7.73940303358924,-1.97221584485231,
0.326719153931175));
#39863=CARTESIAN_POINT('Ctrl Pts',(-7.37994005288748,-2.89008119835739,
0.356422143579367));
#39864=CARTESIAN_POINT('Ctrl Pts',(-6.90067454371506,-4.11385452027366,
0.396024603977074));
#39865=CARTESIAN_POINT('Ctrl Pts',(-6.11045756878819,-5.21593885253046,
0.435627064374781));
#39866=CARTESIAN_POINT('Ctrl Pts',(-5.10512425767101,-6.06252668852639,
0.475229524772489));
#39867=CARTESIAN_POINT('Ctrl Pts',(-4.09979094655382,-6.90911452452231,
0.514831985170196));
#39868=CARTESIAN_POINT('Ctrl Pts',(-2.87934129924631,-7.50020586425735,
0.554434445567904));
#39869=CARTESIAN_POINT('Ctrl Pts',(-1.59182128379852,-7.7641673765801,0.594036905965611));
#39870=CARTESIAN_POINT('Ctrl Pts',(-0.304301268350717,-8.02812888890286,
0.633639366363318));
#39871=CARTESIAN_POINT('Ctrl Pts',(1.05028911523738,-7.96496057381331,0.673241826761026));
#39872=CARTESIAN_POINT('Ctrl Pts',(2.30764556912295,-7.5822916411342,0.712844287158734));
#39873=CARTESIAN_POINT('Ctrl Pts',(3.56500202300852,-7.1996227084551,0.752446747556441));
#39874=CARTESIAN_POINT('Ctrl Pts',(4.72512454719156,-6.49745315818644,0.792049207954148));
#39875=CARTESIAN_POINT('Ctrl Pts',(5.64729088391455,-5.56097129020032,0.831651668351856));
#39876=CARTESIAN_POINT('Ctrl Pts',(6.56945722063754,-4.6244894222142,0.871254128749563));
#39877=CARTESIAN_POINT('Ctrl Pts',(7.25366736990048,-3.45369523651063,0.910856589147271));
#39878=CARTESIAN_POINT('Ctrl Pts',(7.61692939337572,-2.19059467623739,0.950459049544978));
#39879=CARTESIAN_POINT('Ctrl Pts',(7.98019141685096,-0.927494115964165,
0.990061509942686));
#39880=CARTESIAN_POINT('Ctrl Pts',(8.0225053145385,0.427912818878729,1.02966397034039));
#39881=CARTESIAN_POINT('Ctrl Pts',(7.73873794470293,1.71121413696055,1.0692664307381));
#39882=CARTESIAN_POINT('Ctrl Pts',(7.45497057486737,2.99451545504238,1.10886889113581));
#39883=CARTESIAN_POINT('Ctrl Pts',(6.8451219375087,4.20571115636314,1.14847135153352));
#39884=CARTESIAN_POINT('Ctrl Pts',(5.98316549926359,5.19788834344375,1.18807381193122));
#39885=CARTESIAN_POINT('Ctrl Pts',(5.12120906101848,6.19006553052436,1.22767627232893));
#39886=CARTESIAN_POINT('Ctrl Pts',(4.00714482188693,6.9632242033648,1.26727873272664));
#39887=CARTESIAN_POINT('Ctrl Pts',(2.77610595421604,7.42358092802782,1.30688119312434));
#39888=CARTESIAN_POINT('Ctrl Pts',(1.54506708654514,7.88393765269083,1.34648365352205));
#39889=CARTESIAN_POINT('Ctrl Pts',(0.197053590334899,8.03149242917641,1.38608611391976));
#39890=CARTESIAN_POINT('Ctrl Pts',(-1.10442365502742,7.84834779953031,1.42568857431747));
#39891=CARTESIAN_POINT('Ctrl Pts',(-2.40590090038974,7.66520316988421,1.46529103471517));
#39892=CARTESIAN_POINT('Ctrl Pts',(-3.66084189490413,7.15135913410644,1.50489349511288));
#39893=CARTESIAN_POINT('Ctrl Pts',(-4.71702534436858,6.36914344397809,1.54449595551059));
#39894=CARTESIAN_POINT('Ctrl Pts',(-5.77320879383302,5.58692775384975,1.5840984159083));
#39895=CARTESIAN_POINT('Ctrl Pts',(-6.63063469824751,4.53634040937083,1.62370087630601));
#39896=CARTESIAN_POINT('Ctrl Pts',(-7.18529933225044,3.34481528739395,1.66330333670371));
#39897=CARTESIAN_POINT('Ctrl Pts',(-7.67088009423164,2.30169546114194,1.69797328268074));
#39898=CARTESIAN_POINT('Ctrl Pts',(-7.92442114724993,1.15055930628868,1.73264322865776));
#39899=CARTESIAN_POINT('Ctrl Pts',(-7.92542130335282,-0.000150527452605021,
1.76731317463479));
#39900=CARTESIAN_POINT('Origin',(0.,0.,0.));
#39901=CARTESIAN_POINT('',(-7.92433472984446,2.91513625877426E-5,3.4826868253652));
#39902=CARTESIAN_POINT('',(-7.92432847716457,-1.12691906257078E-6,3.26731317463479));
#39903=CARTESIAN_POINT('',(-7.925,-9.70532588324277E-16,0.));
#39904=CARTESIAN_POINT('Ctrl Pts',(-7.92433472984446,2.91513625877426E-5,
3.4826868253652));
#39905=CARTESIAN_POINT('Ctrl Pts',(-7.92441529464847,0.625845985284648,
3.46383890818084));
#39906=CARTESIAN_POINT('Ctrl Pts',(-7.8511761824248,1.25164427548606,3.44499099099648));
#39907=CARTESIAN_POINT('Ctrl Pts',(-7.70440497514907,1.85969334967445,3.42614307381212));
#39908=CARTESIAN_POINT('Ctrl Pts',(-7.39601541322528,3.13730079801299,3.38654061341441));
#39909=CARTESIAN_POINT('Ctrl Pts',(-6.76299144473731,4.33654782151547,3.34693815301671));
#39910=CARTESIAN_POINT('Ctrl Pts',(-5.8821173587817,5.31196863257356,3.307335692619));
#39911=CARTESIAN_POINT('Ctrl Pts',(-5.00124327282608,6.28738944363165,3.26773323222129));
#39912=CARTESIAN_POINT('Ctrl Pts',(-3.87251906940282,7.03898404224534,3.22813077182358));
#39913=CARTESIAN_POINT('Ctrl Pts',(-2.63285628719021,7.47558580627131,3.18852831142588));
#39914=CARTESIAN_POINT('Ctrl Pts',(-1.3931935049776,7.91218757029729,3.14892585102817));
#39915=CARTESIAN_POINT('Ctrl Pts',(-0.0425921439756402,8.03379649973554,
3.10932339063046));
#39916=CARTESIAN_POINT('Ctrl Pts',(1.25512309008608,7.82566172311737,3.06972093023275));
#39917=CARTESIAN_POINT('Ctrl Pts',(2.5528383241478,7.6175269464992,3.03011846983505));
#39918=CARTESIAN_POINT('Ctrl Pts',(3.79766743126929,7.0796484638246,2.99051600943734));
#39919=CARTESIAN_POINT('Ctrl Pts',(4.8386156264262,6.27726964496666,2.95091354903963));
#39920=CARTESIAN_POINT('Ctrl Pts',(5.87956382158311,5.47489082610872,2.91131108864192));
#39921=CARTESIAN_POINT('Ctrl Pts',(6.71663110477544,4.40801167106745,2.87170862824421));
#39922=CARTESIAN_POINT('Ctrl Pts',(7.2482832222225,3.20604206247861,2.83210616784651));
#39923=CARTESIAN_POINT('Ctrl Pts',(7.77993533966956,2.00407245388978,2.7925037074488));
#39924=CARTESIAN_POINT('Ctrl Pts',(8.00617229137134,0.667012391753384,2.7529012470511));
#39925=CARTESIAN_POINT('Ctrl Pts',(7.8995520777056,-0.642955945262401,2.71329878665339));
#39926=CARTESIAN_POINT('Ctrl Pts',(7.79293186403986,-1.9529242822782,2.67369632625568));
#39927=CARTESIAN_POINT('Ctrl Pts',(7.35345448500659,-3.23580089417338,2.63409386585797));
#39928=CARTESIAN_POINT('Ctrl Pts',(6.63442749261576,-4.33597592487487,2.59449140546026));
#39929=CARTESIAN_POINT('Ctrl Pts',(5.91540050022493,-5.43615095557636,2.55488894506255));
#39930=CARTESIAN_POINT('Ctrl Pts',(4.91682389447654,-6.35362440508415,2.51528648466485));
#39931=CARTESIAN_POINT('Ctrl Pts',(3.75982262260237,-6.97710894444533,2.47568402426714));
#39932=CARTESIAN_POINT('Ctrl Pts',(2.60282135072821,-7.60059348380651,2.43608156386943));
#39933=CARTESIAN_POINT('Ctrl Pts',(1.28739541272828,-7.93008911302109,2.39647910347173));
#39934=CARTESIAN_POINT('Ctrl Pts',(-0.0268971801072414,-7.92562880264182,
2.35687664307402));
#39935=CARTESIAN_POINT('Ctrl Pts',(-1.34118977294278,-7.92116849226255,
2.31727418267631));
#39936=CARTESIAN_POINT('Ctrl Pts',(-2.65434902061391,-7.58275224228942,
2.2776717222786));
#39937=CARTESIAN_POINT('Ctrl Pts',(-3.80709185594238,-6.95142913198073,
2.2380692618809));
#39938=CARTESIAN_POINT('Ctrl Pts',(-4.95983469127085,-6.32010602167203,
2.19846680148319));
#39939=CARTESIAN_POINT('Ctrl Pts',(-5.95216111425665,-5.39587605102776,
2.15886434108548));
#39940=CARTESIAN_POINT('Ctrl Pts',(-6.66370430982927,-4.29084609912597,
2.11926188068777));
#39941=CARTESIAN_POINT('Ctrl Pts',(-7.37524750540189,-3.18581614722418,
2.07965942029007));
#39942=CARTESIAN_POINT('Ctrl Pts',(-7.80600747356133,-1.89998621406488,
2.04005695989236));
#39943=CARTESIAN_POINT('Ctrl Pts',(-7.90373406335874,-0.58932438581693,
2.00045449949465));
#39944=CARTESIAN_POINT('Ctrl Pts',(-7.9183490997636,-0.393314575446958,
1.9945319414515));
#39945=CARTESIAN_POINT('Ctrl Pts',(-7.92551575184149,-0.196749392822418,
1.98860938340835));
#39946=CARTESIAN_POINT('Ctrl Pts',(-7.92532948546385,-0.000170658577658411,
1.9826868253652));
#39947=CARTESIAN_POINT('Ctrl Pts',(-7.92542130335282,-0.000150527452605021,
1.76731317463479));
#39948=CARTESIAN_POINT('Ctrl Pts',(-7.92556359617334,-0.163862719352453,
1.77224568905547));
#39949=CARTESIAN_POINT('Ctrl Pts',(-7.92059422714886,-0.327566282117818,
1.77717820347615));
#39950=CARTESIAN_POINT('Ctrl Pts',(-7.91045415923277,-0.490948934636991,
1.78211071789683));
#39951=CARTESIAN_POINT('Ctrl Pts',(-7.82904098862079,-1.80272513521619,
1.82171317829454));
#39952=CARTESIAN_POINT('Ctrl Pts',(-7.41431128380546,-3.09381463689972,
1.86131563869225));
#39953=CARTESIAN_POINT('Ctrl Pts',(-6.71657075814878,-4.20761134022216,
1.90091809908996));
#39954=CARTESIAN_POINT('Ctrl Pts',(-6.01883023249209,-5.3214080435446,1.94052055948766));
#39955=CARTESIAN_POINT('Ctrl Pts',(-5.03807888599404,-6.25791194850595,
1.98012301988537));
#39956=CARTESIAN_POINT('Ctrl Pts',(-3.89327950730805,-6.9035273977777,2.01972548028308));
#39957=CARTESIAN_POINT('Ctrl Pts',(-2.74848012862205,-7.54914284704945,
2.05932794068079));
#39958=CARTESIAN_POINT('Ctrl Pts',(-1.43963271774809,-7.90386984063161,
2.0989304010785));
#39959=CARTESIAN_POINT('Ctrl Pts',(-0.125497325076411,-7.92468083470104,
2.1385328614762));
#39960=CARTESIAN_POINT('Ctrl Pts',(1.18863806759526,-7.94549182877046,2.17813532187391));
#39961=CARTESIAN_POINT('Ctrl Pts',(2.50806144206467,-7.63238682332716,2.21773778227162));
#39962=CARTESIAN_POINT('Ctrl Pts',(3.67272990690861,-7.02334470981914,2.25734024266932));
#39963=CARTESIAN_POINT('Ctrl Pts',(4.83739837175256,-6.41430259631112,2.29694270306703));
#39964=CARTESIAN_POINT('Ctrl Pts',(5.84731192697105,-5.50932337473839,2.33654516346474));
#39965=CARTESIAN_POINT('Ctrl Pts',(6.57997048089828,-4.41817885144047,2.37614762386244));
#39966=CARTESIAN_POINT('Ctrl Pts',(7.31262903482551,-3.32703432814256,2.41575008426015));
#39967=CARTESIAN_POINT('Ctrl Pts',(7.76803258746148,-2.04972450311947,2.45535254465786));
#39968=CARTESIAN_POINT('Ctrl Pts',(7.89094177996011,-0.741183995942706,
2.49495500505557));
#39969=CARTESIAN_POINT('Ctrl Pts',(8.01385097245874,0.567356511234078,2.53455746545328));
#39970=CARTESIAN_POINT('Ctrl Pts',(7.80426580482004,1.90712770056451,2.57415992585098));
#39971=CARTESIAN_POINT('Ctrl Pts',(7.28760845528799,3.11561854086603,2.61376238624869));
#39972=CARTESIAN_POINT('Ctrl Pts',(6.77095110575595,4.32410938116752,2.6533648466464));
#39973=CARTESIAN_POINT('Ctrl Pts',(5.94722157433056,5.40131987244009,2.69296730704411));
#39974=CARTESIAN_POINT('Ctrl Pts',(4.91633627744731,6.21658696537909,2.73256976744181));
#39975=CARTESIAN_POINT('Ctrl Pts',(3.88545098056406,7.03185405831809,2.77217222783952));
#39976=CARTESIAN_POINT('Ctrl Pts',(2.64740991822295,7.58517775292355,2.81177468823723));
#39977=CARTESIAN_POINT('Ctrl Pts',(1.35238450192072,7.80944121234524,2.85137714863493));
#39978=CARTESIAN_POINT('Ctrl Pts',(0.0573590856184794,8.03370467176694,
2.89097960903264));
#39979=CARTESIAN_POINT('Ctrl Pts',(-1.29465068464487,7.92890789600487,2.93058206943035));
#39980=CARTESIAN_POINT('Ctrl Pts',(-2.53964926648632,7.50776248251543,2.97018452982806));
#39981=CARTESIAN_POINT('Ctrl Pts',(-3.78464784832777,7.08661706902599,3.00978699022577));
#39982=CARTESIAN_POINT('Ctrl Pts',(-4.92263524174732,6.34912301780917,3.04938945062347));
#39983=CARTESIAN_POINT('Ctrl Pts',(-5.81557630533137,5.38473658847692,3.08899191102118));
#39984=CARTESIAN_POINT('Ctrl Pts',(-6.70851736891541,4.42035015914468,3.12859437141889));
#39985=CARTESIAN_POINT('Ctrl Pts',(-7.35641210266396,3.229071351697,3.16819683181659));
#39986=CARTESIAN_POINT('Ctrl Pts',(-7.6806724293244,1.95539942822157,3.2077992922143));
#39987=CARTESIAN_POINT('Ctrl Pts',(-7.84310333858861,1.31738215745299,3.22763725302113));
#39988=CARTESIAN_POINT('Ctrl Pts',(-7.92432520227825,0.658690118588125,
3.24747521382796));
#39989=CARTESIAN_POINT('Ctrl Pts',(-7.92432847716457,-1.12691906257078E-6,
3.26731317463479));
#39990=CARTESIAN_POINT('Origin',(0.,0.,0.));
#39991=CARTESIAN_POINT('',(-7.92549788412615,0.000128118915216219,4.9826868253652));
#39992=CARTESIAN_POINT('',(-7.92541478162738,0.000152176599558203,4.76731317463479));
#39993=CARTESIAN_POINT('',(-7.925,-9.70532588324277E-16,0.));
#39994=CARTESIAN_POINT('Ctrl Pts',(-7.92549788412615,0.000128118915216219,
4.9826868253652));
#39995=CARTESIAN_POINT('Ctrl Pts',(-7.9256005347688,0.133414831212393,4.97867089335104));
#39996=CARTESIAN_POINT('Ctrl Pts',(-7.92230720286013,0.266696470636857,
4.97465496133688));
#39997=CARTESIAN_POINT('Ctrl Pts',(-7.91558408688892,0.399804876554018,
4.97063902932271));
#39998=CARTESIAN_POINT('Ctrl Pts',(-7.84928517220114,1.71243177246342,4.931036568925));
#39999=CARTESIAN_POINT('Ctrl Pts',(-7.44945356408088,3.00821240714173,4.89143410852729));
#40000=CARTESIAN_POINT('Ctrl Pts',(-6.76458787761404,4.12997169747715,4.85183164812959));
#40001=CARTESIAN_POINT('Ctrl Pts',(-6.0797221911472,5.2517309878126,4.81222918773188));
#40002=CARTESIAN_POINT('Ctrl Pts',(-5.10982242633376,6.19946893380517,4.77262672733417));
#40003=CARTESIAN_POINT('Ctrl Pts',(-3.97253509838228,6.8582271957151,4.73302426693646));
#40004=CARTESIAN_POINT('Ctrl Pts',(-2.83524777043081,7.51698545762502,4.69342180653876));
#40005=CARTESIAN_POINT('Ctrl Pts',(-1.5305728793413,7.88676403545229,4.65381934614105));
#40006=CARTESIAN_POINT('Ctrl Pts',(-0.216764360195708,7.92270967460465,
4.61421688574334));
#40007=CARTESIAN_POINT('Ctrl Pts',(1.09704415894986,7.95865531375702,4.57461442534563));
#40008=CARTESIAN_POINT('Ctrl Pts',(2.4199863061515,7.66076801423447,4.53501196494793));
#40009=CARTESIAN_POINT('Ctrl Pts',(3.59159237197411,7.0651807909991,4.49540950455022));
#40010=CARTESIAN_POINT('Ctrl Pts',(4.76319843779671,6.46959356776373,4.45580704415251));
#40011=CARTESIAN_POINT('Ctrl Pts',(5.78346842224027,5.57630642081553,4.4162045837548));
#40012=CARTESIAN_POINT('Ctrl Pts',(6.52864602326593,4.4936729385681,4.3766021233571));
#40013=CARTESIAN_POINT('Ctrl Pts',(7.27382362429159,3.41103945632067,4.33699966295939));
#40014=CARTESIAN_POINT('Ctrl Pts',(7.74390884189933,2.13905963877403,4.29739720256168));
#40015=CARTESIAN_POINT('Ctrl Pts',(7.88188146667275,0.832021587007101,4.25779474216397));
#40016=CARTESIAN_POINT('Ctrl Pts',(8.01985409144617,-0.475016464759823,
4.21819228176627));
#40017=CARTESIAN_POINT('Ctrl Pts',(7.82571412338525,-1.81711275074703,4.17858982136856));
#40018=CARTESIAN_POINT('Ctrl Pts',(7.32301027497934,-3.03147421042508,4.13898736097086));
#40019=CARTESIAN_POINT('Ctrl Pts',(6.82030642657341,-4.24583567010315,4.09938490057315));
#40020=CARTESIAN_POINT('Ctrl Pts',(6.00903869782248,-5.33246230347208,4.05978244017544));
#40021=CARTESIAN_POINT('Ctrl Pts',(4.98761191843291,-6.15954890613194,4.02017997977773));
#40022=CARTESIAN_POINT('Ctrl Pts',(3.96618513904335,-6.9866355087918,3.98057751938002));
#40023=CARTESIAN_POINT('Ctrl Pts',(2.73459930901516,-7.55418208074261,3.94097505898231));
#40024=CARTESIAN_POINT('Ctrl Pts',(1.44224283562455,-7.79334658404302,3.90137259858461));
#40025=CARTESIAN_POINT('Ctrl Pts',(0.149886362233948,-8.03251108734343,
3.8617701381869));
#40026=CARTESIAN_POINT('Ctrl Pts',(-1.20324075451908,-7.94329352199344,
3.82216767778919));
#40027=CARTESIAN_POINT('Ctrl Pts',(-2.45300744079018,-7.5365157646855,3.78256521739149));
#40028=CARTESIAN_POINT('Ctrl Pts',(-3.70277412706129,-7.12973800737757,
3.74296275699378));
#40029=CARTESIAN_POINT('Ctrl Pts',(-4.84918038285048,-6.40540005811169,
3.70336029659607));
#40030=CARTESIAN_POINT('Ctrl Pts',(-5.75316987893714,-5.45136237284001,
3.66375783619837));
#40031=CARTESIAN_POINT('Ctrl Pts',(-6.65715937502381,-4.49732468756832,
3.62415537580066));
#40032=CARTESIAN_POINT('Ctrl Pts',(-7.31873211140794,-3.31358726629082,
3.58455291540295));
#40033=CARTESIAN_POINT('Ctrl Pts',(-7.6576409019202,-2.04373461906477,3.54495045500524));
#40034=CARTESIAN_POINT('Ctrl Pts',(-7.83525353172734,-1.37824031954997,
3.5241959117919));
#40035=CARTESIAN_POINT('Ctrl Pts',(-7.92424601523,-0.689094341500147,3.50344136857855));
#40036=CARTESIAN_POINT('Ctrl Pts',(-7.92433472984446,2.91513625877426E-5,
3.4826868253652));
#40037=CARTESIAN_POINT('Ctrl Pts',(-7.92432847716457,-1.12691906257078E-6,
3.26731317463479));
#40038=CARTESIAN_POINT('Ctrl Pts',(-7.92433173992378,-0.656253197336447,
3.28707767422567));
#40039=CARTESIAN_POINT('Ctrl Pts',(-7.84371681523565,-1.31250448026098,
3.30684217381655));
#40040=CARTESIAN_POINT('Ctrl Pts',(-7.68247426549688,-1.94830825344823,
3.32660667340742));
#40041=CARTESIAN_POINT('Ctrl Pts',(-7.35938985543661,-3.22227897213938,
3.36620913380513));
#40042=CARTESIAN_POINT('Ctrl Pts',(-6.71259511574375,-4.4141553700185,3.40581159420284));
#40043=CARTESIAN_POINT('Ctrl Pts',(-5.82054469703419,-5.37936569869396,
3.44541405460055));
#40044=CARTESIAN_POINT('Ctrl Pts',(-4.92849427832463,-6.34457602736943,
3.48501651499825));
#40045=CARTESIAN_POINT('Ctrl Pts',(-3.79118818059835,-7.08312028684125,
3.52461897539596));
#40046=CARTESIAN_POINT('Ctrl Pts',(-2.54657890572889,-7.50541482979923,
3.56422143579367));
#40047=CARTESIAN_POINT('Ctrl Pts',(-1.30196963085945,-7.92770937275721,
3.60382389619138));
#40048=CARTESIAN_POINT('Ctrl Pts',(0.0499428211531797,-8.03375419920136,
3.64342635658908));
#40049=CARTESIAN_POINT('Ctrl Pts',(1.34517471238414,-7.81068632602966,3.68302881698679));
#40050=CARTESIAN_POINT('Ctrl Pts',(2.6404066036151,-7.58761845285795,3.7226312773845));
#40051=CARTESIAN_POINT('Ctrl Pts',(3.87895793406438,-7.0354378800704,3.76223373778221));
#40052=CARTESIAN_POINT('Ctrl Pts',(4.91059539796127,-6.22112278676367,3.80183619817991));
#40053=CARTESIAN_POINT('Ctrl Pts',(5.94223286185817,-5.40680769345693,3.84143865857762));
#40054=CARTESIAN_POINT('Ctrl Pts',(6.76695645920266,-4.33035807963103,3.88104111897533));
#40055=CARTESIAN_POINT('Ctrl Pts',(7.28472919570126,-3.12234470162488,3.92064357937303));
#40056=CARTESIAN_POINT('Ctrl Pts',(7.80250193219985,-1.91433132361873,3.96024603977074));
#40057=CARTESIAN_POINT('Ctrl Pts',(8.01332380785255,-0.574754181432342,
3.99984850016845));
#40058=CARTESIAN_POINT('Ctrl Pts',(7.89162263479,0.733899230506076,4.03945096056616));
#40059=CARTESIAN_POINT('Ctrl Pts',(7.76992146172746,2.0425526424445,4.07905342096387));
#40060=CARTESIAN_POINT('Ctrl Pts',(7.31569723994968,3.32028232413496,4.11865588136157));
#40061=CARTESIAN_POINT('Ctrl Pts',(6.58404627812082,4.41210272976854,4.15825834175928));
#40062=CARTESIAN_POINT('Ctrl Pts',(5.85239531629196,5.50392313540212,4.19786080215699));
#40063=CARTESIAN_POINT('Ctrl Pts',(4.84331761441201,6.40983426497883,4.2374632625547));
#40064=CARTESIAN_POINT('Ctrl Pts',(3.67921187748911,7.01995127127036,4.2770657229524));
#40065=CARTESIAN_POINT('Ctrl Pts',(2.51510614056621,7.63006827756189,4.31666818335011));
#40066=CARTESIAN_POINT('Ctrl Pts',(1.19597236860035,7.94439116056824,4.35627064374782));
#40067=CARTESIAN_POINT('Ctrl Pts',(-0.118181675755223,7.92479330847078,
4.39587310414552));
#40068=CARTESIAN_POINT('Ctrl Pts',(-1.43233572011079,7.90519545637331,4.43547556454323));
#40069=CARTESIAN_POINT('Ctrl Pts',(-2.74151003685607,7.55167686917203,4.47507802494094));
#40070=CARTESIAN_POINT('Ctrl Pts',(-3.88690492136875,6.90711850359517,4.51468048533865));
#40071=CARTESIAN_POINT('Ctrl Pts',(-5.03229980588144,6.26256013801832,4.55428294573635));
#40072=CARTESIAN_POINT('Ctrl Pts',(-6.01391525816152,5.32696199406589,4.59388540613406));
#40073=CARTESIAN_POINT('Ctrl Pts',(-6.71268367821032,4.21380988260697,4.63348786653177));
#40074=CARTESIAN_POINT('Ctrl Pts',(-7.41145209825913,3.10065777114805,4.67309032692948));
#40075=CARTESIAN_POINT('Ctrl Pts',(-7.82737348607664,1.80995169218265,4.71269278732718));
#40076=CARTESIAN_POINT('Ctrl Pts',(-7.90999757489035,0.498251197385663,
4.75229524772489));
#40077=CARTESIAN_POINT('Ctrl Pts',(-7.92044172839613,0.332444814308169,
4.75730122336152));
#40078=CARTESIAN_POINT('Ctrl Pts',(-7.92556032633143,0.166302974182222,
4.76230719899816));
#40079=CARTESIAN_POINT('Ctrl Pts',(-7.92541478162738,0.000152176599558203,
4.76731317463479));
#40080=CARTESIAN_POINT('Origin',(0.,0.,0.));
#40081=CARTESIAN_POINT('',(-7.92482915763566,-0.000199399977182102,6.4826868253652));
#40082=CARTESIAN_POINT('',(-7.92492875745862,-0.000203300716254766,6.26731317463479));
#40083=CARTESIAN_POINT('',(-7.925,-9.70532588324277E-16,0.));
#40084=CARTESIAN_POINT('Ctrl Pts',(-7.92482915763566,-0.000199399977182102,
6.4826868253652));
#40085=CARTESIAN_POINT('Ctrl Pts',(-7.92390949144967,0.955439152281158,
6.45390041812353));
#40086=CARTESIAN_POINT('Ctrl Pts',(-7.75084131112706,1.91140179707541,6.42511401088185));
#40087=CARTESIAN_POINT('Ctrl Pts',(-7.41274235439825,2.80491820972297,6.39632760364018));
#40088=CARTESIAN_POINT('Ctrl Pts',(-6.94760787506061,4.03415977674095,6.35672514324247));
#40089=CARTESIAN_POINT('Ctrl Pts',(-6.17012854586171,5.14521272810185,6.31712268284476));
#40090=CARTESIAN_POINT('Ctrl Pts',(-5.1746107446823,6.0033090056188,6.27752022244705));
#40091=CARTESIAN_POINT('Ctrl Pts',(-4.17909294350288,6.86140528313575,6.23791776204934));
#40092=CARTESIAN_POINT('Ctrl Pts',(-2.96553667034296,7.46654488680876,6.19831530165164));
#40093=CARTESIAN_POINT('Ctrl Pts',(-1.68114339047374,7.74532583411388,6.15871284125393));
#40094=CARTESIAN_POINT('Ctrl Pts',(-0.396750110604525,8.02410678141899,
6.11911038085622));
#40095=CARTESIAN_POINT('Ctrl Pts',(0.958480175973984,7.9765290723562,6.07950792045851));
#40096=CARTESIAN_POINT('Ctrl Pts',(2.22016128596198,7.60836376892173,6.03990546006081));
#40097=CARTESIAN_POINT('Ctrl Pts',(3.48184239594998,7.24019846548726,6.0003029996631));
#40098=CARTESIAN_POINT('Ctrl Pts',(4.64997432934747,6.5514455676811,5.9607005392654));
#40099=CARTESIAN_POINT('Ctrl Pts',(5.58286548434806,5.62564915006263,5.92109807886769));
#40100=CARTESIAN_POINT('Ctrl Pts',(6.51575663934865,4.69985273244416,5.88149561846998));
#40101=CARTESIAN_POINT('Ctrl Pts',(7.21340701595235,3.53701279501336,5.84189315807227));
#40102=CARTESIAN_POINT('Ctrl Pts',(7.59119329676186,2.2781790331585,5.80229069767456));
#40103=CARTESIAN_POINT('Ctrl Pts',(7.96897957757138,1.01934527130364,5.76268823727685));
#40104=CARTESIAN_POINT('Ctrl Pts',(8.02690176258671,-0.335482314975283,
5.72308577687915));
#40105=CARTESIAN_POINT('Ctrl Pts',(7.7579340296894,-1.62196638895895,5.68348331648145));
#40106=CARTESIAN_POINT('Ctrl Pts',(7.48896629679208,-2.90845046294262,5.64388085608374));
#40107=CARTESIAN_POINT('Ctrl Pts',(6.89310864598212,-4.12659102463103,5.60427839568602));
#40108=CARTESIAN_POINT('Ctrl Pts',(6.04263718116354,-5.12863054554968,5.56467593528832));
#40109=CARTESIAN_POINT('Ctrl Pts',(5.19216571634494,-6.13067006646835,5.52507347489061));
#40110=CARTESIAN_POINT('Ctrl Pts',(4.08708043751773,-6.91660854661725,5.48547101449291));
#40111=CARTESIAN_POINT('Ctrl Pts',(2.86142553850362,-7.39111353339431,5.4458685540952));
#40112=CARTESIAN_POINT('Ctrl Pts',(1.63577063948951,-7.86561852017137,5.40626609369749));
#40113=CARTESIAN_POINT('Ctrl Pts',(0.289546120288506,-8.0286900135766,5.36666363329978));
#40114=CARTESIAN_POINT('Ctrl Pts',(-1.01395421378253,-7.86054783257998,
5.32706117290207));
#40115=CARTESIAN_POINT('Ctrl Pts',(-2.31745454785354,-7.69240565158337,
5.28745871250436));
#40116=CARTESIAN_POINT('Ctrl Pts',(-3.57823069679459,-7.19304979618491,
5.24785625210666));
#40117=CARTESIAN_POINT('Ctrl Pts',(-4.64335353765705,-6.42305093396068,
5.20825379170896));
#40118=CARTESIAN_POINT('Ctrl Pts',(-5.70847637851951,-5.65305207173644,
5.16865133131125));
#40119=CARTESIAN_POINT('Ctrl Pts',(-6.57794591130339,-4.61241020268642,
5.12904887091354));
#40120=CARTESIAN_POINT('Ctrl Pts',(-7.14629756706768,-3.42735268959116,
5.08944641051583));
#40121=CARTESIAN_POINT('Ctrl Pts',(-7.65701488428923,-2.36246726574673,
5.05385988213228));
#40122=CARTESIAN_POINT('Ctrl Pts',(-7.92458826215163,-1.1809704040634,5.01827335374875));
#40123=CARTESIAN_POINT('Ctrl Pts',(-7.92549788412615,0.000128118915216219,
4.9826868253652));
#40124=CARTESIAN_POINT('Ctrl Pts',(-7.92541478162738,0.000152176599558203,
4.76731317463479));
#40125=CARTESIAN_POINT('Ctrl Pts',(-7.92440891673685,-1.14812219664027,
4.80190965939586));
#40126=CARTESIAN_POINT('Ctrl Pts',(-7.67197476697247,-2.29682439984853,
4.83650614415694));
#40127=CARTESIAN_POINT('Ctrl Pts',(-7.18838400348709,-3.33818083825282,
4.87110262891801));
#40128=CARTESIAN_POINT('Ctrl Pts',(-6.63481955346023,-4.53021746846575,
4.91070508931572));
#40129=CARTESIAN_POINT('Ctrl Pts',(-5.77836386359658,-5.58159581826305,
4.95030754971343));
#40130=CARTESIAN_POINT('Ctrl Pts',(-4.7229029549041,-6.36478621550053,4.98991001011114));
#40131=CARTESIAN_POINT('Ctrl Pts',(-3.66744204621164,-7.14797661273799,
5.02951247050884));
#40132=CARTESIAN_POINT('Ctrl Pts',(-2.41297591869036,-7.66297905741564,
5.06911493090655));
#40133=CARTESIAN_POINT('Ctrl Pts',(-1.11166830482495,-7.84732498820554,
5.10871739130425));
#40134=CARTESIAN_POINT('Ctrl Pts',(0.189639309040495,-8.03167091899544,
5.14831985170196));
#40135=CARTESIAN_POINT('Ctrl Pts',(1.53778840925007,-7.88536033589756,5.18792231209968));
#40136=CARTESIAN_POINT('Ctrl Pts',(2.76925174342659,-7.42614036172198,5.22752477249738));
#40137=CARTESIAN_POINT('Ctrl Pts',(4.0007150776031,-6.96692038754639,5.26712723289509));
#40138=CARTESIAN_POINT('Ctrl Pts',(5.11549264574657,-6.1947910222931,5.30672969329279));
#40139=CARTESIAN_POINT('Ctrl Pts',(5.97836460258773,-5.20340970604791,5.3463321536905));
#40140=CARTESIAN_POINT('Ctrl Pts',(6.84123655942888,-4.21202838980272,5.38593461408821));
#40141=CARTESIAN_POINT('Ctrl Pts',(7.45220290496774,-3.00139512256563,5.42553707448592));
#40142=CARTESIAN_POINT('Ctrl Pts',(7.73715488686723,-1.71835681600012,5.46513953488363));
#40143=CARTESIAN_POINT('Ctrl Pts',(8.02210686876671,-0.435318509434607,
5.50474199528134));
#40144=CARTESIAN_POINT('Ctrl Pts',(7.98104448702682,0.920124836459304,5.54434445567904));
#40145=CARTESIAN_POINT('Ctrl Pts',(7.61894851006622,2.1835611947979,5.58394691607674));
#40146=CARTESIAN_POINT('Ctrl Pts',(7.25685253310561,3.44699755313651,5.62354937647445));
#40147=CARTESIAN_POINT('Ctrl Pts',(6.57372296092429,4.61842692391978,5.66315183687216));
#40148=CARTESIAN_POINT('Ctrl Pts',(5.65242177217065,5.5557577340952,5.70275429726987));
#40149=CARTESIAN_POINT('Ctrl Pts',(4.73112058341702,6.4930885442706,5.74235675766758));
#40150=CARTESIAN_POINT('Ctrl Pts',(3.57164777809107,7.19632079383816,5.78195921806528));
#40151=CARTESIAN_POINT('Ctrl Pts',(2.31464462653267,7.58015409759795,5.82156167846299));
#40152=CARTESIAN_POINT('Ctrl Pts',(1.05764147497426,7.96398740135773,5.8611641388607));
#40153=CARTESIAN_POINT('Ctrl Pts',(-0.296892022816619,8.02842175930975,
5.90076659925841));
#40154=CARTESIAN_POINT('Ctrl Pts',(-1.58465420234887,7.76564143837748,5.94036905965612));
#40155=CARTESIAN_POINT('Ctrl Pts',(-2.87241638188114,7.50286111744522,5.97997152005382));
#40156=CARTESIAN_POINT('Ctrl Pts',(-4.09340724315476,6.91286611762868,6.01957398045153));
#40157=CARTESIAN_POINT('Ctrl Pts',(-5.09952352319192,6.06722141732769,6.05917644084924));
#40158=CARTESIAN_POINT('Ctrl Pts',(-6.10563980322905,5.22157671702672,6.09877890124694));
#40159=CARTESIAN_POINT('Ctrl Pts',(-6.8968815020297,4.12028231624131,6.13838136164465));
#40160=CARTESIAN_POINT('Ctrl Pts',(-7.37727289928889,2.896922584379,6.17798382204235));
#40161=CARTESIAN_POINT('Ctrl Pts',(-7.73847143827851,1.97709814470656,6.2077602729065));
#40162=CARTESIAN_POINT('Ctrl Pts',(-7.92393718090885,0.98826659176352,6.23753672377064));
#40163=CARTESIAN_POINT('Ctrl Pts',(-7.92492875745862,-0.000203300716254766,
6.26731317463479));
#40164=CARTESIAN_POINT('Origin',(0.,0.,0.));
#40165=CARTESIAN_POINT('',(-7.92455486516943,0.000157560269493928,7.9826868253652));
#40166=CARTESIAN_POINT('',(-7.92448697665393,0.000136394684465916,7.76731317463479));
#40167=CARTESIAN_POINT('',(-7.925,-9.70532588324277E-16,0.));
#40168=CARTESIAN_POINT('Ctrl Pts',(-7.92455486516943,0.000157560269493928,
7.9826868253652));
#40169=CARTESIAN_POINT('Ctrl Pts',(-7.92488905702959,0.463456370592923,
7.96873240329372));
#40170=CARTESIAN_POINT('Ctrl Pts',(-7.88492338787207,0.926698172538998,
7.95477798122224));
#40171=CARTESIAN_POINT('Ctrl Pts',(-7.80412960742409,1.38270620395372,7.94082355915076));
#40172=CARTESIAN_POINT('Ctrl Pts',(-7.57483795534541,2.67685080647717,7.90122109875306));
#40173=CARTESIAN_POINT('Ctrl Pts',(-7.01670987890586,3.9127334135031,7.86161863835535));
#40174=CARTESIAN_POINT('Ctrl Pts',(-6.19744497513114,4.94044442901112,7.82201617795764));
#40175=CARTESIAN_POINT('Ctrl Pts',(-5.37818007135641,5.96815544451915,7.78241371755994));
#40176=CARTESIAN_POINT('Ctrl Pts',(-4.2977783402465,6.78769486850925,7.74281125716223));
#40177=CARTESIAN_POINT('Ctrl Pts',(-3.08728992048746,7.29965453448188,7.70320879676452));
#40178=CARTESIAN_POINT('Ctrl Pts',(-1.87680150072842,7.8116142004545,7.66360633636682));
#40179=CARTESIAN_POINT('Ctrl Pts',(-0.536226392320244,8.01599410840963,
7.62400387596911));
#40180=CARTESIAN_POINT('Ctrl Pts',(0.771826859399493,7.88800346570884,7.5844014155714));
#40181=CARTESIAN_POINT('Ctrl Pts',(2.07988011111925,7.76001282300805,7.54479895517369));
#40182=CARTESIAN_POINT('Ctrl Pts',(3.35541150615052,7.29965162965135,7.50519649477599));
#40183=CARTESIAN_POINT('Ctrl Pts',(4.44370214558388,6.56276059423613,7.46559403437828));
#40184=CARTESIAN_POINT('Ctrl Pts',(5.53199278501721,5.82586955882093,7.42599157398057));
#40185=CARTESIAN_POINT('Ctrl Pts',(6.43304266885262,4.81244868134719,7.38638911358286));
#40186=CARTESIAN_POINT('Ctrl Pts',(7.03755660731061,3.64542348360573,7.34678665318516));
#40187=CARTESIAN_POINT('Ctrl Pts',(7.64207054576862,2.47839828586421,7.30718419278745));
#40188=CARTESIAN_POINT('Ctrl Pts',(7.95004853884922,1.15776876785491,7.26758173238974));
#40189=CARTESIAN_POINT('Ctrl Pts',(7.92413359466385,-0.156275877361342,
7.22797927199203));
#40190=CARTESIAN_POINT('Ctrl Pts',(7.89821865047848,-1.47032052257757,7.18837681159432));
#40191=CARTESIAN_POINT('Ctrl Pts',(7.53841076902715,-2.77778029500072,7.14877435119662));
#40192=CARTESIAN_POINT('Ctrl Pts',(6.88835378334602,-3.92006346012254,7.10917189079891));
#40193=CARTESIAN_POINT('Ctrl Pts',(6.23829679766489,-5.06234662524434,7.0695694304012));
#40194=CARTESIAN_POINT('Ctrl Pts',(5.29799070775395,-6.0394531830648,7.0299669700035));
#40195=CARTESIAN_POINT('Ctrl Pts',(4.18149238703527,-6.73286245166878,6.99036450960579));
#40196=CARTESIAN_POINT('Ctrl Pts',(3.06499406631659,-7.42627172027276,6.95076204920808));
#40197=CARTESIAN_POINT('Ctrl Pts',(1.77230351479016,-7.83598369966026,6.91115958881037));
#40198=CARTESIAN_POINT('Ctrl Pts',(0.460220995892857,-7.91230130940832,
6.87155712841267));
#40199=CARTESIAN_POINT('Ctrl Pts',(-0.851861523004442,-7.98861891915639,
6.83195466801496));
#40200=CARTESIAN_POINT('Ctrl Pts',(-2.18333600927261,-7.73154215926501,
6.79235220761725));
#40201=CARTESIAN_POINT('Ctrl Pts',(-3.37269780121221,-7.17225382412137,
6.75274974721954));
#40202=CARTESIAN_POINT('Ctrl Pts',(-4.56205959315182,-6.61296548897771,
6.71314728682183));
#40203=CARTESIAN_POINT('Ctrl Pts',(-5.60930869076286,-5.75146557858178,
6.67354482642413));
#40204=CARTESIAN_POINT('Ctrl Pts',(-6.38741629028751,-4.69225196579373,
6.63394236602643));
#40205=CARTESIAN_POINT('Ctrl Pts',(-7.16552388981217,-3.63303835300566,
6.59433990562872));
#40206=CARTESIAN_POINT('Ctrl Pts',(-7.67448999125043,-2.37611103782545,
6.554737445231));
#40207=CARTESIAN_POINT('Ctrl Pts',(-7.85257822723136,-1.07393228889779,
6.51513498483329));
#40208=CARTESIAN_POINT('Ctrl Pts',(-7.90121691804727,-0.71828684602346,
6.50431893167726));
#40209=CARTESIAN_POINT('Ctrl Pts',(-7.92517470816823,-0.359266000140281,
6.49350287852123));
#40210=CARTESIAN_POINT('Ctrl Pts',(-7.92482915763566,-0.000199399977182102,
6.4826868253652));
#40211=CARTESIAN_POINT('Ctrl Pts',(-7.92492875745862,-0.000203300716254766,
6.26731317463479));
#40212=CARTESIAN_POINT('Ctrl Pts',(-7.92525597041882,-0.326391086878601,
6.27713918416835));
#40213=CARTESIAN_POINT('Ctrl Pts',(-7.90549484318086,-0.652539489974055,
6.28696519370192));
#40214=CARTESIAN_POINT('Ctrl Pts',(-7.86533125816864,-0.976155771249044,
6.29679120323548));
#40215=CARTESIAN_POINT('Ctrl Pts',(-7.70345712407144,-2.28044933207546,
6.33639366363319));
#40216=CARTESIAN_POINT('Ctrl Pts',(-7.2101677601593,-3.54361139078904,6.3759961240309));
#40217=CARTESIAN_POINT('Ctrl Pts',(-6.44529798314124,-4.61242341930822,
6.4155985844286));
#40218=CARTESIAN_POINT('Ctrl Pts',(-5.68042820612317,-5.68123544782742,
6.45520104482631));
#40219=CARTESIAN_POINT('Ctrl Pts',(-4.64397801599918,-6.55569744615223,
6.49480350522402));
#40220=CARTESIAN_POINT('Ctrl Pts',(-3.4616663349496,-7.12973927124577,6.53440596562173));
#40221=CARTESIAN_POINT('Ctrl Pts',(-2.27935465390004,-7.70378109633929,
6.57400842601944));
#40222=CARTESIAN_POINT('Ctrl Pts',(-0.951181481924927,-7.97740274820154,
6.61361088641714));
#40223=CARTESIAN_POINT('Ctrl Pts',(0.361748960782006,-7.91741457673151,
6.65321334681485));
#40224=CARTESIAN_POINT('Ctrl Pts',(1.67467940348893,-7.85742640526148,6.69281580721256));
#40225=CARTESIAN_POINT('Ctrl Pts',(2.97236711692768,-7.46382841045917,6.73241826761026));
#40226=CARTESIAN_POINT('Ctrl Pts',(4.09740569390686,-6.78436308506606,6.77202072800797));
#40227=CARTESIAN_POINT('Ctrl Pts',(5.22244427088606,-6.10489775967295,6.81162318840568));
#40228=CARTESIAN_POINT('Ctrl Pts',(6.1748337114057,-5.13956510368905,6.85122564880339));
#40229=CARTESIAN_POINT('Ctrl Pts',(6.8390514605963,-4.00545765297588,6.89082810920109));
#40230=CARTESIAN_POINT('Ctrl Pts',(7.5032692097869,-2.87135020226273,6.9304305695988));
#40231=CARTESIAN_POINT('Ctrl Pts',(7.87931526764847,-1.56846795682031,6.97003302999651));
#40232=CARTESIAN_POINT('Ctrl Pts',(7.92157614929286,-0.254847408113207,
7.00963549039422));
#40233=CARTESIAN_POINT('Ctrl Pts',(7.96383703093724,1.05877314059392,7.04923795079192));
#40234=CARTESIAN_POINT('Ctrl Pts',(7.67231273636446,2.38313199256569,7.08884041118962));
#40235=CARTESIAN_POINT('Ctrl Pts',(7.08236446329754,3.5575875954764,7.12844287158733));
#40236=CARTESIAN_POINT('Ctrl Pts',(6.49241619023065,4.73204319838707,7.16804533198504));
#40237=CARTESIAN_POINT('Ctrl Pts',(5.60404393866961,5.75659555223666,7.20764779238275));
#40238=CARTESIAN_POINT('Ctrl Pts',(4.52500513200579,6.50696891384835,7.24725025278046));
#40239=CARTESIAN_POINT('Ctrl Pts',(3.44596632534194,7.25734227546006,7.28685271317817));
#40240=CARTESIAN_POINT('Ctrl Pts',(2.17626096357527,7.73353664483391,7.32645517357588));
#40241=CARTESIAN_POINT('Ctrl Pts',(0.869901261753817,7.87779078709676,7.36605763397359));
#40242=CARTESIAN_POINT('Ctrl Pts',(-0.436458440067604,8.0220449293596,7.40566009437129));
#40243=CARTESIAN_POINT('Ctrl Pts',(-1.7794724819438,7.83435884451148,7.445262554769));
#40244=CARTESIAN_POINT('Ctrl Pts',(-2.99623648175723,7.33749840448736,7.48486501516671));
#40245=CARTESIAN_POINT('Ctrl Pts',(-4.21300048157064,6.84063796446325,7.52446747556441));
#40246=CARTESIAN_POINT('Ctrl Pts',(-5.30351443932127,6.03460316926317,7.56406993596212));
#40247=CARTESIAN_POINT('Ctrl Pts',(-6.13550162748532,5.01716410630472,7.60367239635983));
#40248=CARTESIAN_POINT('Ctrl Pts',(-6.9674888156494,3.99972504334623,7.64327485675754));
#40249=CARTESIAN_POINT('Ctrl Pts',(-7.54094923422687,2.77088171262934,7.68287731715525));
#40250=CARTESIAN_POINT('Ctrl Pts',(-7.78632350986467,1.47968986284162,7.72247977755296));
#40251=CARTESIAN_POINT('Ctrl Pts',(-7.87891844986639,0.992443057727118,
7.7374242432469));
#40252=CARTESIAN_POINT('Ctrl Pts',(-7.92479322829447,0.496317691455577,
7.75236870894085));
#40253=CARTESIAN_POINT('Ctrl Pts',(-7.92448697665393,0.000136394684465916,
7.76731317463479));
#40254=CARTESIAN_POINT('Origin',(0.,0.,0.));
#40255=CARTESIAN_POINT('',(-7.92566451523509,-3.0530117057781E-5,9.4826868253652));
#40256=CARTESIAN_POINT('',(-7.92567438502354,3.93182477014807E-6,9.2673131746348));
#40257=CARTESIAN_POINT('',(-7.925,-9.70532588324277E-16,0.));
#40258=CARTESIAN_POINT('Ctrl Pts',(-7.92566451523509,-3.0530117057781E-5,
9.4826868253652));
#40259=CARTESIAN_POINT('Ctrl Pts',(-7.92538377707008,1.28515034464984,9.44396192806621));
#40260=CARTESIAN_POINT('Ctrl Pts',(-7.60662215046401,2.57046545380378,9.40523703076722));
#40261=CARTESIAN_POINT('Ctrl Pts',(-7.00560821546851,3.70644963641561,9.36651213346824));
#40262=CARTESIAN_POINT('Ctrl Pts',(-6.39097442121051,4.86817689051166,9.32690967307053));
#40263=CARTESIAN_POINT('Ctrl Pts',(-5.48115086564248,5.8737284137033,9.28730721267282));
#40264=CARTESIAN_POINT('Ctrl Pts',(-4.38649696388181,6.60113321799984,9.24770475227511));
#40265=CARTESIAN_POINT('Ctrl Pts',(-3.29184306212112,7.32853802229639,9.2081022918774));
#40266=CARTESIAN_POINT('Ctrl Pts',(-2.01235881416776,7.77779610769788,9.1684998314797));
#40267=CARTESIAN_POINT('Ctrl Pts',(-0.703242590509952,7.89441354597149,
9.12889737108199));
#40268=CARTESIAN_POINT('Ctrl Pts',(0.60587363314786,8.01103098424511,9.08929491068428));
#40269=CARTESIAN_POINT('Ctrl Pts',(1.94462183251012,7.79500777539085,9.04969245028657));
#40270=CARTESIAN_POINT('Ctrl Pts',(3.15061506192477,7.27254701652028,9.01008998988886));
#40271=CARTESIAN_POINT('Ctrl Pts',(4.35660829133941,6.75008625764971,8.97048752949116));
#40272=CARTESIAN_POINT('Ctrl Pts',(5.42984655080643,5.92118794876284,8.93088506909345));
#40273=CARTESIAN_POINT('Ctrl Pts',(6.24014861356879,4.88639546665032,8.89128260869575));
#40274=CARTESIAN_POINT('Ctrl Pts',(7.05045067633115,3.85160298453779,8.85168014829804));
#40275=CARTESIAN_POINT('Ctrl Pts',(7.59781654238885,2.61091632919961,8.81207768790033));
#40276=CARTESIAN_POINT('Ctrl Pts',(7.81585204502282,1.31482781619415,8.77247522750262));
#40277=CARTESIAN_POINT('Ctrl Pts',(8.03388754765679,0.0187393031886965,
8.73287276710491));
#40278=CARTESIAN_POINT('Ctrl Pts',(7.92259268686704,-1.33275106748403,8.69327030670721));
#40279=CARTESIAN_POINT('Ctrl Pts',(7.49546726233136,-2.57571075535358,8.6536678463095));
#40280=CARTESIAN_POINT('Ctrl Pts',(7.06834183779569,-3.81867044322313,8.6140653859118));
#40281=CARTESIAN_POINT('Ctrl Pts',(6.32538584951409,-4.95309944828949,8.57446292551408));
#40282=CARTESIAN_POINT('Ctrl Pts',(5.35671807691682,-5.84139425311781,8.53486046511638));
#40283=CARTESIAN_POINT('Ctrl Pts',(4.38805030431956,-6.72968905794612,8.49525800471867));
#40284=CARTESIAN_POINT('Ctrl Pts',(3.19367074740664,-7.3718496625364,8.45565554432097));
#40285=CARTESIAN_POINT('Ctrl Pts',(1.91845478176303,-7.68998352574672,8.41605308392326));
#40286=CARTESIAN_POINT('Ctrl Pts',(0.643238816119382,-8.00811738895705,
8.37645062352555));
#40287=CARTESIAN_POINT('Ctrl Pts',(-0.712813558254954,-8.00222451078741,
8.33684816312784));
#40288=CARTESIAN_POINT('Ctrl Pts',(-1.98521644078227,-7.67301968322596,
8.29724570273013));
#40289=CARTESIAN_POINT('Ctrl Pts',(-3.25761932330957,-7.34381485566452,
8.25764324233242));
#40290=CARTESIAN_POINT('Ctrl Pts',(-4.44637271398986,-6.69129807871128,
8.21804078193472));
#40291=CARTESIAN_POINT('Ctrl Pts',(-5.40728367770804,-5.79461807237694,
8.17843832153702));
#40292=CARTESIAN_POINT('Ctrl Pts',(-6.36819464142624,-4.89793806604258,
8.13883586113931));
#40293=CARTESIAN_POINT('Ctrl Pts',(-7.10126317818233,-3.75709483032712,
8.0992334007416));
#40294=CARTESIAN_POINT('Ctrl Pts',(-7.51756983270146,-2.51046991345888,
8.05963094034389));
#40295=CARTESIAN_POINT('Ctrl Pts',(-7.78718563241042,-1.70310887262521,
8.03398290201766));
#40296=CARTESIAN_POINT('Ctrl Pts',(-7.92394062506736,-0.851379363495959,
8.00833486369143));
#40297=CARTESIAN_POINT('Ctrl Pts',(-7.92455486516943,0.000157560269493928,
7.9826868253652));
#40298=CARTESIAN_POINT('Ctrl Pts',(-7.92448697665393,0.000136394684465916,
7.76731317463479));
#40299=CARTESIAN_POINT('Ctrl Pts',(-7.92398166910498,-0.818550337812214,
7.79197116933855));
#40300=CARTESIAN_POINT('Ctrl Pts',(-7.7977523179122,-1.63738933647875,7.81662916404231));
#40301=CARTESIAN_POINT('Ctrl Pts',(-7.54822065908196,-2.41675004340037,
7.84128715874607));
#40302=CARTESIAN_POINT('Ctrl Pts',(-7.1474553999633,-3.6684577309962,7.88088961914378));
#40303=CARTESIAN_POINT('Ctrl Pts',(-6.42863674902783,-4.81833273732931,
7.92049207954149));
#40304=CARTESIAN_POINT('Ctrl Pts',(-5.47895568457806,-5.72689798205777,
7.9600945399392));
#40305=CARTESIAN_POINT('Ctrl Pts',(-4.52927462012827,-6.63546322678623,
7.9996970003369));
#40306=CARTESIAN_POINT('Ctrl Pts',(-3.34873114216419,-7.30271870991004,
8.03929946073461));
#40307=CARTESIAN_POINT('Ctrl Pts',(-2.08052234307956,-7.64772794171015,
8.07890192113232));
#40308=CARTESIAN_POINT('Ctrl Pts',(-0.812313543994936,-7.99273717351026,
8.11850438153002));
#40309=CARTESIAN_POINT('Ctrl Pts',(0.543560576210242,-8.01550015398668,
8.15810684192774));
#40310=CARTESIAN_POINT('Ctrl Pts',(1.82263573876145,-7.71325578820364,8.19770930232545));
#40311=CARTESIAN_POINT('Ctrl Pts',(3.10171090131263,-7.41101142242061,8.23731176272315));
#40312=CARTESIAN_POINT('Ctrl Pts',(4.30398710620981,-6.78375971037817,8.27691422312085));
#40313=CARTESIAN_POINT('Ctrl Pts',(5.28363113340734,-5.90758478031049,8.31651668351856));
#40314=CARTESIAN_POINT('Ctrl Pts',(6.26327516060488,-5.0314098502428,8.35611914391626));
#40315=CARTESIAN_POINT('Ctrl Pts',(7.02028701010276,-3.90631170214984,8.39572160431398));
#40316=CARTESIAN_POINT('Ctrl Pts',(7.46284296021754,-2.66876204289534,8.43532406471169));
#40317=CARTESIAN_POINT('Ctrl Pts',(7.90539891033232,-1.43121238364084,8.4749265251094));
#40318=CARTESIAN_POINT('Ctrl Pts',(8.03349896106404,-0.0812112132247506,
8.51452898550711));
#40319=CARTESIAN_POINT('Ctrl Pts',(7.83160488350145,1.21748956430181,8.55413144590481));
#40320=CARTESIAN_POINT('Ctrl Pts',(7.62971080593885,2.51619034182838,8.59373390630252));
#40321=CARTESIAN_POINT('Ctrl Pts',(7.09782260008196,3.76359072646538,8.63333636670022));
#40322=CARTESIAN_POINT('Ctrl Pts',(6.30045702958997,4.80838404339315,8.67293882709792));
#40323=CARTESIAN_POINT('Ctrl Pts',(5.50309145909799,5.8531773603209,8.71254128749563));
#40324=CARTESIAN_POINT('Ctrl Pts',(4.44024852397089,6.69536360953942,8.75214374789334));
#40325=CARTESIAN_POINT('Ctrl Pts',(3.2408485230561,7.23278761896632,8.79174620829105));
#40326=CARTESIAN_POINT('Ctrl Pts',(2.04144852214128,7.77021162839325,8.83134866868876));
#40327=CARTESIAN_POINT('Ctrl Pts',(0.705491455438782,8.00287339802857,8.87095112908646));
#40328=CARTESIAN_POINT('Ctrl Pts',(-0.604974289096646,7.9025516132449,8.91055358948417));
#40329=CARTESIAN_POINT('Ctrl Pts',(-1.91544003363207,7.80222982846123,8.95015604988188));
#40330=CARTESIAN_POINT('Ctrl Pts',(-3.20041445600039,7.36892448925854,8.98975851027959));
#40331=CARTESIAN_POINT('Ctrl Pts',(-4.30403324072476,6.65519449401772,9.0293609706773));
#40332=CARTESIAN_POINT('Ctrl Pts',(-5.40765202544913,5.94146449877691,9.06896343107501));
#40333=CARTESIAN_POINT('Ctrl Pts',(-6.32991517252957,4.94730984749797,9.10856589147271));
#40334=CARTESIAN_POINT('Ctrl Pts',(-6.95895437423414,3.79331911494341,9.14816835187042));
#40335=CARTESIAN_POINT('Ctrl Pts',(-7.58799357593871,2.63932838238885,9.18777081226812));
#40336=CARTESIAN_POINT('Ctrl Pts',(-7.9238088322674,1.32550156855867,9.22737327266583));
#40337=CARTESIAN_POINT('Ctrl Pts',(-7.92566655806616,0.0112027148127723,
9.26697573306354));
#40338=CARTESIAN_POINT('Ctrl Pts',(-7.92567183445477,0.00746978958662008,
9.26708821358729));
#40339=CARTESIAN_POINT('Ctrl Pts',(-7.92567441681873,0.00373686055253689,
9.26720069411104));
#40340=CARTESIAN_POINT('Ctrl Pts',(-7.92567430608102,3.93136451648719E-6,
9.2673131746348));
#40341=CARTESIAN_POINT('Origin',(0.,0.,0.));
#40342=CARTESIAN_POINT('',(-7.92444197974487,-0.000117952357666096,10.9826868253652));
#40343=CARTESIAN_POINT('',(-7.92450147625162,-0.000141486819805631,10.7673131746348));
#40344=CARTESIAN_POINT('',(-7.925,-9.70532588324277E-16,0.));
#40345=CARTESIAN_POINT('Ctrl Pts',(-7.92444197974487,-0.000117952357666096,
10.9826868253652));
#40346=CARTESIAN_POINT('Ctrl Pts',(-7.92402168439202,0.79317964478778,10.9587939132364));
#40347=CARTESIAN_POINT('Ctrl Pts',(-7.80562445932409,1.58659993568632,10.9349010011076));
#40348=CARTESIAN_POINT('Ctrl Pts',(-7.57110679996587,2.34406851422498,10.9110080889788));
#40349=CARTESIAN_POINT('Ctrl Pts',(-7.18239418648314,3.5995713688952,10.8714056285811));
#40350=CARTESIAN_POINT('Ctrl Pts',(-6.47466384601646,4.75630406628582,10.8318031681834));
#40351=CARTESIAN_POINT('Ctrl Pts',(-5.53376177138355,5.67395770459255,10.7922007077857));
#40352=CARTESIAN_POINT('Ctrl Pts',(-4.59285969675065,6.59161134289928,10.752598247388));
#40353=CARTESIAN_POINT('Ctrl Pts',(-3.41878588795152,7.27018592212212,10.7129957869903));
#40354=CARTESIAN_POINT('Ctrl Pts',(-2.15395268203755,7.62737197332591,10.6733933265926));
#40355=CARTESIAN_POINT('Ctrl Pts',(-0.889119476123588,7.98455802452969,
10.6337908661949));
#40356=CARTESIAN_POINT('Ctrl Pts',(0.46647312690522,8.02035554771443,10.5941884057972));
#40357=CARTESIAN_POINT('Ctrl Pts',(1.74839499563781,7.73042238918058,10.5545859453995));
#40358=CARTESIAN_POINT('Ctrl Pts',(3.0303168643704,7.44048923064672,10.5149834850018));
#40359=CARTESIAN_POINT('Ctrl Pts',(4.23856799880677,6.82482539039427,10.475381024604));
#40360=CARTESIAN_POINT('Ctrl Pts',(5.22659043427609,5.95810941560032,10.4357785642063));
#40361=CARTESIAN_POINT('Ctrl Pts',(6.21461286974541,5.09139344080638,10.3961761038086));
#40362=CARTESIAN_POINT('Ctrl Pts',(6.98240660624767,3.97362533147094,10.3565736434109));
#40363=CARTESIAN_POINT('Ctrl Pts',(7.43684010506711,2.74038767833817,10.3169711830132));
#40364=CARTESIAN_POINT('Ctrl Pts',(7.89127360388654,1.5071500252054,10.2773687226155));
#40365=CARTESIAN_POINT('Ctrl Pts',(8.03234686502314,0.158442828275303,10.2377662622178));
#40366=CARTESIAN_POINT('Ctrl Pts',(7.84294804025856,-1.14213896428184,10.1981638018201));
#40367=CARTESIAN_POINT('Ctrl Pts',(7.65354921549399,-2.442720756839,10.1585613414224));
#40368=CARTESIAN_POINT('Ctrl Pts',(7.13367830482823,-3.69517714502321,10.1189588810247));
#40369=CARTESIAN_POINT('Ctrl Pts',(6.34639440283714,-4.7475881729108,10.079356420627));
#40370=CARTESIAN_POINT('Ctrl Pts',(5.55911050084605,-5.79999920079838,10.0397539602293));
#40371=CARTESIAN_POINT('Ctrl Pts',(4.50441360752963,-6.65236486838934,10.0001514998316));
#40372=CARTESIAN_POINT('Ctrl Pts',(3.31023592640137,-7.20129526456781,9.96054903943384));
#40373=CARTESIAN_POINT('Ctrl Pts',(2.11605824527312,-7.75022566074628,9.92094657903614));
#40374=CARTESIAN_POINT('Ctrl Pts',(0.782399776333046,-7.99572078551226,
9.88134411863843));
#40375=CARTESIAN_POINT('Ctrl Pts',(-0.52896990685943,-7.90800266904119,
9.84174165824072));
#40376=CARTESIAN_POINT('Ctrl Pts',(-1.84033959005191,-7.82028455257012,
9.80213919784301));
#40377=CARTESIAN_POINT('Ctrl Pts',(-3.12942048749678,-7.39935319486198,
9.76253673744531));
#40378=CARTESIAN_POINT('Ctrl Pts',(-4.23985017813971,-6.69626656002088,
9.7229342770476));
#40379=CARTESIAN_POINT('Ctrl Pts',(-5.35027986878263,-5.99317992517977,
9.68333181664989));
#40380=CARTESIAN_POINT('Ctrl Pts',(-6.28205835262362,-5.0079380132057,9.64372935625218));
#40381=CARTESIAN_POINT('Ctrl Pts',(-6.92216313440376,-3.86004830496029,
9.60412689585448));
#40382=CARTESIAN_POINT('Ctrl Pts',(-7.56226791618391,-2.71215859671488,
9.56452443545677));
#40383=CARTESIAN_POINT('Ctrl Pts',(-7.91069899590321,-1.40162109219814,
9.52492197505906));
#40384=CARTESIAN_POINT('Ctrl Pts',(-7.92519251928886,-0.0874008474395132,
9.48531951466136));
#40385=CARTESIAN_POINT('Ctrl Pts',(-7.92551368573069,-0.058278636879719,
9.48444195156264));
#40386=CARTESIAN_POINT('Ctrl Pts',(-7.92567087717459,-0.0291546179659009,
9.48356438846392));
#40387=CARTESIAN_POINT('Ctrl Pts',(-7.92566451523509,-3.0530117057781E-5,
9.4826868253652));
#40388=CARTESIAN_POINT('Ctrl Pts',(-7.92567430608102,3.93136451648719E-6,
9.2673131746348));
#40389=CARTESIAN_POINT('Ctrl Pts',(-7.9256354279719,-1.31056338809906,9.30680315450875));
#40390=CARTESIAN_POINT('Ctrl Pts',(-7.59364712907968,-2.62114968173378,
9.34629313438271));
#40391=CARTESIAN_POINT('Ctrl Pts',(-6.96965005365923,-3.77363141019302,
9.38578311425666));
#40392=CARTESIAN_POINT('Ctrl Pts',(-6.34387562818474,-4.92939578779125,
9.42538557465437));
#40393=CARTESIAN_POINT('Ctrl Pts',(-5.42442658196696,-5.92615364932607,
9.46498803505207));
#40394=CARTESIAN_POINT('Ctrl Pts',(-4.32282987905268,-6.64300065687463,
9.50459049544978));
#40395=CARTESIAN_POINT('Ctrl Pts',(-3.22123317613842,-7.35984766442319,
9.54419295584749));
#40396=CARTESIAN_POINT('Ctrl Pts',(-1.93748881652769,-7.7967838179855,9.5837954162452));
#40397=CARTESIAN_POINT('Ctrl Pts',(-0.627311912035025,-7.90080981010722,
9.6233978766429));
#40398=CARTESIAN_POINT('Ctrl Pts',(0.682864992457676,-8.00483580222894,
9.66300033704061));
#40399=CARTESIAN_POINT('Ctrl Pts',(2.01947444183229,-7.77595163291006,9.70260279743832));
#40400=CARTESIAN_POINT('Ctrl Pts',(3.22038891568058,-7.24192040292001,9.74220525783603));
#40401=CARTESIAN_POINT('Ctrl Pts',(4.42130338952884,-6.70788917292997,9.78180771823373));
#40402=CARTESIAN_POINT('Ctrl Pts',(5.48652288785077,-5.86871088226878,9.82141017863144));
#40403=CARTESIAN_POINT('Ctrl Pts',(6.28683884038356,-4.82617584486022,9.86101263902915));
#40404=CARTESIAN_POINT('Ctrl Pts',(7.08715479291634,-3.78364080745165,9.90061509942685));
#40405=CARTESIAN_POINT('Ctrl Pts',(7.62256719965997,-2.53774902329572,9.94021755982456));
#40406=CARTESIAN_POINT('Ctrl Pts',(7.82813181984032,-1.2396241775921,9.97982002022227));
#40407=CARTESIAN_POINT('Ctrl Pts',(8.03369644002068,0.0585006681115341,
10.01942248062));
#40408=CARTESIAN_POINT('Ctrl Pts',(7.90941327363775,1.40885857536285,10.0590249410177));
#40409=CARTESIAN_POINT('Ctrl Pts',(7.47035757068589,2.64765436878824,10.0986274014154));
#40410=CARTESIAN_POINT('Ctrl Pts',(7.03130186773404,3.8864501622136,10.1382298618131));
#40411=CARTESIAN_POINT('Ctrl Pts',(6.27747362821324,5.01368384181308,10.1778323222108));
#40412=CARTESIAN_POINT('Ctrl Pts',(5.30031040955247,5.89262466587319,10.2174347826085));
#40413=CARTESIAN_POINT('Ctrl Pts',(4.32314719089171,6.77156548993329,10.2570372430062));
#40414=CARTESIAN_POINT('Ctrl Pts',(3.12264899309097,7.40221345845408,10.2966397034039));
#40415=CARTESIAN_POINT('Ctrl Pts',(1.84443336819958,7.70807248543627,10.3362421638016));
#40416=CARTESIAN_POINT('Ctrl Pts',(0.566217743308195,8.01393151241845,10.3758446241993));
#40417=CARTESIAN_POINT('Ctrl Pts',(-0.789715308673824,7.99500159786202,
10.415447084597));
#40418=CARTESIAN_POINT('Ctrl Pts',(-2.05889436068869,7.65357889500015,10.4550495449948));
#40419=CARTESIAN_POINT('Ctrl Pts',(-3.32807341270356,7.31215619213827,10.4946520053925));
#40420=CARTESIAN_POINT('Ctrl Pts',(-4.51049846475127,6.64824070097095,10.5342544657902));
#40421=CARTESIAN_POINT('Ctrl Pts',(-5.4627441940148,5.74236377820361,10.5738569261879));
#40422=CARTESIAN_POINT('Ctrl Pts',(-6.41498992327833,4.83648685543627,10.6134593865856));
#40423=CARTESIAN_POINT('Ctrl Pts',(-7.13705632975766,3.68864850106897,10.6530618469833));
#40424=CARTESIAN_POINT('Ctrl Pts',(-7.54135849019206,2.43807875444513,10.692664307381));
#40425=CARTESIAN_POINT('Ctrl Pts',(-7.79538898898431,1.6523227343239,10.7175472631323));
#40426=CARTESIAN_POINT('Ctrl Pts',(-7.92397123184249,0.826009999126394,
10.7424302188835));
#40427=CARTESIAN_POINT('Ctrl Pts',(-7.92450147625162,-0.000141486819805631,
10.7673131746348));
#40428=CARTESIAN_POINT('Origin',(0.,0.,0.));
#40429=CARTESIAN_POINT('',(-7.92500786703747,0.000202977126703835,12.4826868253652));
#40430=CARTESIAN_POINT('',(-7.92490579193458,0.000202837437923534,12.2673131746348));
#40431=CARTESIAN_POINT('',(-7.925,-9.70532588324277E-16,0.));
#40432=CARTESIAN_POINT('Ctrl Pts',(-7.92500786703747,0.000202977126703835,
12.4826868253652));
#40433=CARTESIAN_POINT('Ctrl Pts',(-7.92531493217766,0.300984151116678,
12.4736258984066));
#40434=CARTESIAN_POINT('Ctrl Pts',(-7.90851822812937,0.601731230547898,
12.464564971448));
#40435=CARTESIAN_POINT('Ctrl Pts',(-7.87435266312157,0.900492052656451,
12.4555040444894));
#40436=CARTESIAN_POINT('Ctrl Pts',(-7.72502572986527,2.20628159052614,12.4159015840917));
#40437=CARTESIAN_POINT('Ctrl Pts',(-7.24390335415058,3.47412787300641,12.376299123694));
#40438=CARTESIAN_POINT('Ctrl Pts',(-6.48934464920618,4.5502440932928,12.3366966632963));
#40439=CARTESIAN_POINT('Ctrl Pts',(-5.73478594426178,5.62636031357918,12.2970942028986));
#40440=CARTESIAN_POINT('Ctrl Pts',(-4.70679091008767,6.51074647167168,12.2574917425009));
#40441=CARTESIAN_POINT('Ctrl Pts',(-3.5300528159044,7.09612869556788,12.2178892821032));
#40442=CARTESIAN_POINT('Ctrl Pts',(-2.35331472172112,7.68151091946408,12.1782868217055));
#40443=CARTESIAN_POINT('Ctrl Pts',(-1.02783356752869,7.96788920916399,12.1386843613077));
#40444=CARTESIAN_POINT('Ctrl Pts',(0.285612929694432,7.92052654057446,12.09908190091));
#40445=CARTESIAN_POINT('Ctrl Pts',(1.59905942691756,7.87316387198493,12.0594794405123));
#40446=CARTESIAN_POINT('Ctrl Pts',(2.90047126717137,7.49206024510598,12.0198769801146));
#40447=CARTESIAN_POINT('Ctrl Pts',(4.03199033200069,6.82344262828845,11.9802745197169));
#40448=CARTESIAN_POINT('Ctrl Pts',(5.16350939683,6.15482501147092,11.9406720593192));
#40449=CARTESIAN_POINT('Ctrl Pts',(6.12513568623482,5.19869340471483,11.9010695989215));
#40450=CARTESIAN_POINT('Ctrl Pts',(6.80022622936098,4.0710242723093,11.8614671385238));
#40451=CARTESIAN_POINT('Ctrl Pts',(7.47531677248716,2.94335513990372,11.8218646781261));
#40452=CARTESIAN_POINT('Ctrl Pts',(7.86387156933467,1.64414848184864,11.7822622177284));
#40453=CARTESIAN_POINT('Ctrl Pts',(7.91875985925233,0.330994952927389,11.7426597573307));
#40454=CARTESIAN_POINT('Ctrl Pts',(7.97364814916999,-0.982158575993826,
11.703057296933));
#40455=CARTESIAN_POINT('Ctrl Pts',(7.69486993215784,-2.30925897578126,11.6634548365353));
#40456=CARTESIAN_POINT('Ctrl Pts',(7.11624033511875,-3.48933215259594,11.6238523761376));
#40457=CARTESIAN_POINT('Ctrl Pts',(6.53761073807967,-4.66940532941062,11.5842499157399));
#40458=CARTESIAN_POINT('Ctrl Pts',(5.65912976101366,-5.70245128325254,11.5446474553421));
#40459=CARTESIAN_POINT('Ctrl Pts',(4.58735504055451,-6.46316401678891,11.5050449949444));
#40460=CARTESIAN_POINT('Ctrl Pts',(3.51558032009535,-7.22387675032529,11.4654425345467));
#40461=CARTESIAN_POINT('Ctrl Pts',(2.25051185624305,-7.71225626355612,11.425840074149));
#40462=CARTESIAN_POINT('Ctrl Pts',(0.945599418880597,-7.86906329331735,
11.3862376137513));
#40463=CARTESIAN_POINT('Ctrl Pts',(-0.35931301848186,-8.02587032307857,
11.3466351533536));
#40464=CARTESIAN_POINT('Ctrl Pts',(-1.70406942935446,-7.85110486937019,
11.3070326929559));
#40465=CARTESIAN_POINT('Ctrl Pts',(-2.92555408614859,-7.36596556233821,
11.2674302325582));
#40466=CARTESIAN_POINT('Ctrl Pts',(-4.14703874294271,-6.88082625530622,
11.2278277721605));
#40467=CARTESIAN_POINT('Ctrl Pts',(-5.24525164565834,-6.08531309495062,
11.1882253117628));
#40468=CARTESIAN_POINT('Ctrl Pts',(-6.08698220336153,-5.07591991973112,
11.1486228513651));
#40469=CARTESIAN_POINT('Ctrl Pts',(-6.92871276106471,-4.06652674451163,
11.1090203909674));
#40470=CARTESIAN_POINT('Ctrl Pts',(-7.51396097375545,-2.84325355442823,
11.0694179305697));
#40471=CARTESIAN_POINT('Ctrl Pts',(-7.77173763685142,-1.55448045341163,
11.029815470172));
#40472=CARTESIAN_POINT('Ctrl Pts',(-7.87399277178087,-1.04324849876091,
11.014105921903));
#40473=CARTESIAN_POINT('Ctrl Pts',(-7.92471832321012,-0.521709746057469,
10.9983963736341));
#40474=CARTESIAN_POINT('Ctrl Pts',(-7.92444197974487,-0.000117952357666096,
10.9826868253652));
#40475=CARTESIAN_POINT('Ctrl Pts',(-7.92450147625162,-0.000141486819805631,
10.7673131746348));
#40476=CARTESIAN_POINT('Ctrl Pts',(-7.92481514216503,-0.488851138422702,
10.7820326792812));
#40477=CARTESIAN_POINT('Ctrl Pts',(-7.88031944032983,-0.977504363908973,
10.7967521839277));
#40478=CARTESIAN_POINT('Ctrl Pts',(-7.7904753919032,-1.45767247988534,10.8114716885741));
#40479=CARTESIAN_POINT('Ctrl Pts',(-7.54875221879049,-2.74955282871158,
10.8510741489718));
#40480=CARTESIAN_POINT('Ctrl Pts',(-6.97876795817564,-3.98001238748372,
10.8906766093695));
#40481=CARTESIAN_POINT('Ctrl Pts',(-6.14966033378676,-4.9997993629268,10.9302790697672));
#40482=CARTESIAN_POINT('Ctrl Pts',(-5.32055270939788,-6.01958633836991,
10.9698815301649));
#40483=CARTESIAN_POINT('Ctrl Pts',(-4.23232172123497,-6.82870073048396,
11.0094839905627));
#40484=CARTESIAN_POINT('Ctrl Pts',(-3.01696717808935,-7.32899890413347,
11.0490864509604));
#40485=CARTESIAN_POINT('Ctrl Pts',(-1.80161263494375,-7.82929707778297,
11.0886889113581));
#40486=CARTESIAN_POINT('Ctrl Pts',(-0.459134536815433,-8.02077903296795,
11.1282913717558));
#40487=CARTESIAN_POINT('Ctrl Pts',(0.847627742874828,-7.88021846778281,
11.1678938321535));
#40488=CARTESIAN_POINT('Ctrl Pts',(2.15439002256511,-7.73965790259767,11.2074962925512));
#40489=CARTESIAN_POINT('Ctrl Pts',(3.42543648381735,-7.26705481704241,11.2470987529489));
#40490=CARTESIAN_POINT('Ctrl Pts',(4.50659223942145,-6.51973483188231,11.2867012133466));
#40491=CARTESIAN_POINT('Ctrl Pts',(5.58774799502555,-5.77241484672221,11.3263036737443));
#40492=CARTESIAN_POINT('Ctrl Pts',(6.47901304498153,-4.75037796195727,11.365906134142));
#40493=CARTESIAN_POINT('Ctrl Pts',(7.07227907641263,-3.57759480038614,11.4055085945397));
#40494=CARTESIAN_POINT('Ctrl Pts',(7.66554510784373,-2.40481163881498,11.4451110549374));
#40495=CARTESIAN_POINT('Ctrl Pts',(7.96081212074994,-1.08128220043768,11.4847135153351));
#40496=CARTESIAN_POINT('Ctrl Pts',(7.92226493460879,0.232452568277466,11.5243159757329));
#40497=CARTESIAN_POINT('Ctrl Pts',(7.88371774846763,1.54618733699257,11.5639184361306));
#40498=CARTESIAN_POINT('Ctrl Pts',(7.5113563632791,2.85012743604553,11.6035208965283));
#40499=CARTESIAN_POINT('Ctrl Pts',(6.85034732205659,3.98610805890958,11.643123356926));
#40500=CARTESIAN_POINT('Ctrl Pts',(6.18933828083405,5.12208868177365,11.6827258173237));
#40501=CARTESIAN_POINT('Ctrl Pts',(5.23968158357755,6.09010982844884,11.7223282777214));
#40502=CARTESIAN_POINT('Ctrl Pts',(4.11656830979056,6.77275285551553,11.7619307381191));
#40503=CARTESIAN_POINT('Ctrl Pts',(2.99345503600359,7.45539588258221,11.8015331985168));
#40504=CARTESIAN_POINT('Ctrl Pts',(1.69688518568615,7.85266079004038,11.8411356589145));
#40505=CARTESIAN_POINT('Ctrl Pts',(0.384129572232522,7.91636029760581,11.8807381193122));
#40506=CARTESIAN_POINT('Ctrl Pts',(-0.928626041221122,7.98005980517125,
11.9203405797099));
#40507=CARTESIAN_POINT('Ctrl Pts',(-2.25756741781097,7.71019391284396,11.9599430401076));
#40508=CARTESIAN_POINT('Ctrl Pts',(-3.44149715658974,7.1394967057732,11.9995455005053));
#40509=CARTESIAN_POINT('Ctrl Pts',(-4.62542689536849,6.56879949870245,12.0391479609031));
#40510=CARTESIAN_POINT('Ctrl Pts',(-5.66434499633619,5.69727097688824,12.0787504213008));
#40511=CARTESIAN_POINT('Ctrl Pts',(-6.43223318442422,4.63062546034554,12.1183528816985));
#40512=CARTESIAN_POINT('Ctrl Pts',(-7.20012137251226,3.56397994380283,12.1579553420962));
#40513=CARTESIAN_POINT('Ctrl Pts',(-7.69697964772063,2.3022174325316,12.1975578024939));
#40514=CARTESIAN_POINT('Ctrl Pts',(-7.86254029535431,0.99838669160568,12.2371602628916));
#40515=CARTESIAN_POINT('Ctrl Pts',(-7.90455902808044,0.667478856887011,
12.2472112334727));
#40516=CARTESIAN_POINT('Ctrl Pts',(-7.92523797810166,0.333861292895049,
12.2572622040537));
#40517=CARTESIAN_POINT('Ctrl Pts',(-7.92490579193458,0.000202837437923534,
12.2673131746348));
#40518=CARTESIAN_POINT('Origin',(0.,0.,0.));
#40519=CARTESIAN_POINT('',(-7.92471172241511,-8.01339879119567E-6,13.9826868253652));
#40520=CARTESIAN_POINT('',(-7.92543898861653,-0.000149382597450273,13.7673131746348));
#40521=CARTESIAN_POINT('',(-7.925,-9.70532588324277E-16,0.));
#40522=CARTESIAN_POINT('Ctrl Pts',(-7.92471172241511,-8.01339879119567E-6,
13.9826868253652));
#40523=CARTESIAN_POINT('Ctrl Pts',(-7.92378999755476,1.12304350898084,13.9488554231791));
#40524=CARTESIAN_POINT('Ctrl Pts',(-7.68313346855731,2.24612491945329,13.915024020993));
#40525=CARTESIAN_POINT('Ctrl Pts',(-7.22018928937337,3.2688662481316,13.8811926188069));
#40526=CARTESIAN_POINT('Ctrl Pts',(-6.67827475619426,4.46606974396276,13.8415901584092));
#40527=CARTESIAN_POINT('Ctrl Pts',(-5.83176739335577,5.52578080862963,13.8019876980115));
#40528=CARTESIAN_POINT('Ctrl Pts',(-4.78383316777566,6.31911976065525,13.7623852376138));
#40529=CARTESIAN_POINT('Ctrl Pts',(-3.73589894219555,7.11245871268087,13.722782777216));
#40530=CARTESIAN_POINT('Ctrl Pts',(-2.48653785387384,7.63942555206525,13.6831803168183));
#40531=CARTESIAN_POINT('Ctrl Pts',(-1.18708642259866,7.83625609708293,13.6435778564206));
#40532=CARTESIAN_POINT('Ctrl Pts',(0.112365008676521,8.03308664210061,13.6039753960229));
#40533=CARTESIAN_POINT('Ctrl Pts',(1.46190678290515,7.89978089275159,13.5643729356252));
#40534=CARTESIAN_POINT('Ctrl Pts',(2.69774006309914,7.45243063459268,13.5247704752275));
#40535=CARTESIAN_POINT('Ctrl Pts',(3.93357334329316,7.00508037643375,13.4851680148298));
#40536=CARTESIAN_POINT('Ctrl Pts',(5.05569812945251,6.2436856094649,13.4455655544321));
#40537=CARTESIAN_POINT('Ctrl Pts',(5.92805547631356,5.26064132126167,13.4059630940344));
#40538=CARTESIAN_POINT('Ctrl Pts',(6.80041282317456,4.27759703305851,13.3663606336367));
#40539=CARTESIAN_POINT('Ctrl Pts',(7.42300273073732,3.07290322362089,13.326758173239));
#40540=CARTESIAN_POINT('Ctrl Pts',(7.72027995804387,1.79266613693959,13.2871557128413));
#40541=CARTESIAN_POINT('Ctrl Pts',(8.01755718535043,0.512429050258223,13.2475532524436));
#40542=CARTESIAN_POINT('Ctrl Pts',(7.98952173240083,-0.843351313666888,
13.2079507920459));
#40543=CARTESIAN_POINT('Ctrl Pts',(7.63958780389822,-2.11021171993848,13.1683483316481));
#40544=CARTESIAN_POINT('Ctrl Pts',(7.2896538753956,-3.3770721262101,13.1287458712504));
#40545=CARTESIAN_POINT('Ctrl Pts',(6.61782147133996,-4.55501257482813,13.0891434108527));
#40546=CARTESIAN_POINT('Ctrl Pts',(5.70557531991554,-5.50115698955477,13.049540950455));
#40547=CARTESIAN_POINT('Ctrl Pts',(4.79332916849116,-6.44730140428135,13.0099384900573));
#40548=CARTESIAN_POINT('Ctrl Pts',(3.64066926969804,-7.16164978511656,12.9703360296596));
#40549=CARTESIAN_POINT('Ctrl Pts',(2.38741404450885,-7.55755069275904,12.9307335692619));
#40550=CARTESIAN_POINT('Ctrl Pts',(1.13415881931962,-7.95345160040152,12.8911311088642));
#40551=CARTESIAN_POINT('Ctrl Pts',(-0.219691732265668,-8.03090503485126,
12.8515286484665));
#40552=CARTESIAN_POINT('Ctrl Pts',(-1.50992059338783,-7.78051745619478,
12.8119261880688));
#40553=CARTESIAN_POINT('Ctrl Pts',(-2.80014945451003,-7.5301298775383,12.7723237276711));
#40554=CARTESIAN_POINT('Ctrl Pts',(-4.0267566251691,-6.95190128577559,12.7327212672734));
#40555=CARTESIAN_POINT('Ctrl Pts',(-5.04095667418956,-6.11596871951397,
12.6931188068757));
#40556=CARTESIAN_POINT('Ctrl Pts',(-6.05515672321,-5.28003615325238,12.653516346478));
#40557=CARTESIAN_POINT('Ctrl Pts',(-6.85694965059184,-4.18639961249191,
12.6139138860802));
#40558=CARTESIAN_POINT('Ctrl Pts',(-7.34908036888381,-2.96771494548212,
12.5743114256825));
#40559=CARTESIAN_POINT('Ctrl Pts',(-7.72861302009243,-2.02786176122485,
12.5437698922434));
#40560=CARTESIAN_POINT('Ctrl Pts',(-7.92397284707874,-1.01363570905215,
12.5132283588043));
#40561=CARTESIAN_POINT('Ctrl Pts',(-7.92500786703747,0.000202977126703835,
12.4826868253652));
#40562=CARTESIAN_POINT('Ctrl Pts',(-7.92490579193458,0.000202837437923534,
12.2673131746348));
#40563=CARTESIAN_POINT('Ctrl Pts',(-7.92392911052309,-0.980807341544247,
12.2968646644514));
#40564=CARTESIAN_POINT('Ctrl Pts',(-7.74132045846664,-1.96217100913998,
12.3264161542681));
#40565=CARTESIAN_POINT('Ctrl Pts',(-7.38543284899398,-2.87605590061804,
12.3559676440847));
#40566=CARTESIAN_POINT('Ctrl Pts',(-6.908501734941,-4.10076878133526,12.3955701044824));
#40567=CARTESIAN_POINT('Ctrl Pts',(-6.12037648677604,-5.20429557218911,
12.4351725648801));
#40568=CARTESIAN_POINT('Ctrl Pts',(-5.11665481600748,-6.05278112504653,
12.4747750252778));
#40569=CARTESIAN_POINT('Ctrl Pts',(-4.11293314523893,-6.90126667790396,
12.5143774856755));
#40570=CARTESIAN_POINT('Ctrl Pts',(-2.89361505186678,-7.49471099276496,
12.5539799460733));
#40571=CARTESIAN_POINT('Ctrl Pts',(-1.60660087812754,-7.76113068811402,
12.593582406471));
#40572=CARTESIAN_POINT('Ctrl Pts',(-0.319586704388297,-8.02755038346307,
12.6331848668687));
#40573=CARTESIAN_POINT('Ctrl Pts',(1.03512354971804,-7.96694545930018,12.6727873272664));
#40574=CARTESIAN_POINT('Ctrl Pts',(2.29320674430343,-7.58666716612938,12.7123897876641));
#40575=CARTESIAN_POINT('Ctrl Pts',(3.55128993888883,-7.20638887295857,12.7519922480618));
#40576=CARTESIAN_POINT('Ctrl Pts',(4.71274607395329,-6.50643721077984,12.7915947084595));
#40577=CARTESIAN_POINT('Ctrl Pts',(5.63669337513792,-5.5717146010451,12.8311971688572));
#40578=CARTESIAN_POINT('Ctrl Pts',(6.56064067632253,-4.6369919913104,12.8707996292549));
#40579=CARTESIAN_POINT('Ctrl Pts',(7.24707914362734,-3.46749843401971,12.9104020896526));
#40580=CARTESIAN_POINT('Ctrl Pts',(7.61274530193707,-2.20509076394141,12.9500045500503));
#40581=CARTESIAN_POINT('Ctrl Pts',(7.97841146024682,-0.942683093863061,
12.989607010448));
#40582=CARTESIAN_POINT('Ctrl Pts',(8.02330530956146,0.412638689002901,13.0292094708457));
#40583=CARTESIAN_POINT('Ctrl Pts',(7.74198159896325,1.69647744267076,13.0688119312434));
#40584=CARTESIAN_POINT('Ctrl Pts',(7.46065788836505,2.98031619633858,13.1084143916412));
#40585=CARTESIAN_POINT('Ctrl Pts',(6.85311661785402,4.1926719208083,13.1480168520389));
#40586=CARTESIAN_POINT('Ctrl Pts',(5.99305056654226,5.18648850098789,13.1876193124366));
#40587=CARTESIAN_POINT('Ctrl Pts',(5.13298451523049,6.18030508116749,13.2272217728343));
#40588=CARTESIAN_POINT('Ctrl Pts',(4.02039368311798,6.95558251705697,13.266824233232));
#40589=CARTESIAN_POINT('Ctrl Pts',(2.79023368812278,7.41828205099748,13.3064266936297));
#40590=CARTESIAN_POINT('Ctrl Pts',(1.56007369312757,7.88098158493798,13.3460291540274));
#40591=CARTESIAN_POINT('Ctrl Pts',(0.212344535249671,8.03110321692952,13.3856316144251));
#40592=CARTESIAN_POINT('Ctrl Pts',(-1.08947946657793,7.85043650322858,13.4252340748228));
#40593=CARTESIAN_POINT('Ctrl Pts',(-2.39130346840553,7.66976978952763,13.4648365352205));
#40594=CARTESIAN_POINT('Ctrl Pts',(-3.64722231418283,7.15831473013422,13.5044389956182));
#40595=CARTESIAN_POINT('Ctrl Pts',(-4.70489215064052,6.37811165393581,13.5440414560159));
#40596=CARTESIAN_POINT('Ctrl Pts',(-5.7625619870982,5.59790857773741,13.5836439164136));
#40597=CARTESIAN_POINT('Ctrl Pts',(-6.62198281423625,4.54895748473401,13.6232463768114));
#40598=CARTESIAN_POINT('Ctrl Pts',(-7.17891660675418,3.35848959671542,13.6628488372091));
#40599=CARTESIAN_POINT('Ctrl Pts',(-7.66861446088681,2.31174117166319,13.6976702830176));
#40600=CARTESIAN_POINT('Ctrl Pts',(-7.92445227138459,1.15558268908939,13.7324917288262));
#40601=CARTESIAN_POINT('Ctrl Pts',(-7.92543898861653,-0.000149382597450273,
13.7673131746348));
#40602=CARTESIAN_POINT('Origin',(0.,0.,-2.77281266907387));
#40603=CARTESIAN_POINT('',(-7.06850701680182,0.000181040229527252,12.9771873309261));
#40604=CARTESIAN_POINT('',(-7.06889154461022,-0.000133237967543387,13.2728126690739));
#40605=CARTESIAN_POINT('',(-7.0685,-3.68825033525048E-13,-2.77281266907387));
#40606=CARTESIAN_POINT('',(2.93403320825987,6.43108807842,14.));
#40607=CARTESIAN_POINT('Ctrl Pts',(-7.06850701680181,0.000181040229526898,
12.9771873309261));
#40608=CARTESIAN_POINT('Ctrl Pts',(-7.06758385735974,-0.904086310338917,
13.0077288643652));
#40609=CARTESIAN_POINT('Ctrl Pts',(-6.66739692335297,-2.98168855062559,
13.077872858202));
#40610=CARTESIAN_POINT('Ctrl Pts',(-4.68560277486572,-5.6848334937073,13.1876193124366));
#40611=CARTESIAN_POINT('Ctrl Pts',(-1.40348058465622,-7.23204187258727,
13.3064266936297));
#40612=CARTESIAN_POINT('Ctrl Pts',(2.21911599220716,-7.02479407394702,13.4252340748228));
#40613=CARTESIAN_POINT('Ctrl Pts',(5.30337207849841,-5.11336005630641,13.5440414560159));
#40614=CARTESIAN_POINT('Ctrl Pts',(7.10104299890235,-1.96145896063838,13.6628488372091));
#40615=CARTESIAN_POINT('Ctrl Pts',(7.1760595033216,1.66630135572941,13.7816562184022));
#40616=CARTESIAN_POINT('Ctrl Pts',(5.60022245538124,4.71550133998197,13.8940399393325));
#40617=CARTESIAN_POINT('Ctrl Pts',(3.82727142929074,6.0224930120962,13.9668211998651));
#40618=CARTESIAN_POINT('Ctrl Pts',(2.93403320825987,6.43108807842,14.));
#40619=CARTESIAN_POINT('',(7.03625248964568,-0.674420604634066,14.));
#40620=CARTESIAN_POINT('Origin',(0.,0.,14.));
#40621=CARTESIAN_POINT('Ctrl Pts',(-7.06889154461022,-0.000133237967543647,
13.2728126690739));
#40622=CARTESIAN_POINT('Ctrl Pts',(-7.06901237995171,-0.141666470630141,
13.277593683663));
#40623=CARTESIAN_POINT('Ctrl Pts',(-7.03035435797223,-1.4554918851001,13.3219771586498));
#40624=CARTESIAN_POINT('Ctrl Pts',(-6.25050664162124,-3.89909682044781,
13.4059630940344));
#40625=CARTESIAN_POINT('Ctrl Pts',(-3.63108720070629,-6.40999851148318,
13.5247704752275));
#40626=CARTESIAN_POINT('Ctrl Pts',(-0.130578947762305,-7.3657578324409,
13.6435778564207));
#40627=CARTESIAN_POINT('Ctrl Pts',(3.40120320632095,-6.5348310696329,13.7623852376137));
#40628=CARTESIAN_POINT('Ctrl Pts',(6.10869718244117,-4.11816204547854,13.8811926188069));
#40629=CARTESIAN_POINT('Ctrl Pts',(6.9243752846715,-1.84163918696265,13.9603975396023));
#40630=CARTESIAN_POINT('Ctrl Pts',(7.03625248964568,-0.674420604634066,
14.));
#40631=CARTESIAN_POINT('Origin',(0.,0.,-2.77281266907387));
#40632=CARTESIAN_POINT('',(-7.06800228818001,-0.000105204573031335,11.4771873309261));
#40633=CARTESIAN_POINT('',(-7.06841597353811,0.000180915637408435,11.7728126690739));
#40634=CARTESIAN_POINT('',(-7.0685,-3.68825033525048E-13,-2.77281266907387));
#40635=CARTESIAN_POINT('Ctrl Pts',(-7.06800228818001,-0.000105204573031432,
11.4771873309261));
#40636=CARTESIAN_POINT('Ctrl Pts',(-7.06824876562911,-0.465325594953699,
11.492896879195));
#40637=CARTESIAN_POINT('Ctrl Pts',(-6.90895070021522,-2.10316120251506,
11.5482088878617));
#40638=CARTESIAN_POINT('Ctrl Pts',(-5.65789011484937,-4.71810105207384,
11.643123356926));
#40639=CARTESIAN_POINT('Ctrl Pts',(-2.71932182355139,-6.84671358480829,
11.7619307381191));
#40640=CARTESIAN_POINT('Ctrl Pts',(0.878940898310958,-7.31434624457016,
11.8807381193122));
#40641=CARTESIAN_POINT('Ctrl Pts',(4.26397677341757,-6.00755359247974,11.9995455005054));
#40642=CARTESIAN_POINT('Ctrl Pts',(6.61459233924385,-3.24335725504188,12.1183528816985));
#40643=CARTESIAN_POINT('Ctrl Pts',(7.36053952925658,0.307661991354685,12.2371602628916));
#40644=CARTESIAN_POINT('Ctrl Pts',(6.32085514508631,3.78404392036229,12.3559676440847));
#40645=CARTESIAN_POINT('Ctrl Pts',(3.74776160818102,6.3424349345032,12.4747750252778));
#40646=CARTESIAN_POINT('Ctrl Pts',(0.265479112470959,7.36218168021696,12.593582406471));
#40647=CARTESIAN_POINT('Ctrl Pts',(-3.28120740049152,6.59589842189123,12.7123897876641));
#40648=CARTESIAN_POINT('Ctrl Pts',(-6.03188862411031,4.22948193287789,12.8311971688572));
#40649=CARTESIAN_POINT('Ctrl Pts',(-6.98832057332378,1.70910717488751,12.9194630166112));
#40650=CARTESIAN_POINT('Ctrl Pts',(-7.06878089565903,0.268455075352352,
12.9681264039675));
#40651=CARTESIAN_POINT('Ctrl Pts',(-7.06850701680181,0.000181040229526898,
12.9771873309261));
#40652=CARTESIAN_POINT('Ctrl Pts',(-7.06841597353811,0.000180915637408539,
11.7728126690739));
#40653=CARTESIAN_POINT('Ctrl Pts',(-7.06754484766335,-0.874805891950531,
11.8023641588905));
#40654=CARTESIAN_POINT('Ctrl Pts',(-6.68640271942718,-2.92311539223316,
11.8715181091049));
#40655=CARTESIAN_POINT('Ctrl Pts',(-4.75596440127724,-5.62609998399613,
11.9802745197169));
#40656=CARTESIAN_POINT('Ctrl Pts',(-1.49334612632416,-7.21402218195007,
12.09908190091));
#40657=CARTESIAN_POINT('Ctrl Pts',(2.13155081922184,-7.05185717004641,12.2178892821032));
#40658=CARTESIAN_POINT('Ctrl Pts',(5.23934363589174,-5.17894550161347,12.3366966632963));
#40659=CARTESIAN_POINT('Ctrl Pts',(7.07609706408506,-2.04964636860042,12.4555040444894));
#40660=CARTESIAN_POINT('Ctrl Pts',(7.19622280814078,1.5768868890101,12.5743114256825));
#40661=CARTESIAN_POINT('Ctrl Pts',(5.57058035869953,4.82087544613853,12.6931188068757));
#40662=CARTESIAN_POINT('Ctrl Pts',(2.5935399939851,6.89534177632834,12.8119261880688));
#40663=CARTESIAN_POINT('Ctrl Pts',(-1.01267712366536,7.29703316651084,12.9307335692619));
#40664=CARTESIAN_POINT('Ctrl Pts',(-4.37323069894997,5.92849559402285,13.049540950455));
#40665=CARTESIAN_POINT('Ctrl Pts',(-6.58030514877926,3.23468938944454,13.163567317059));
#40666=CARTESIAN_POINT('Ctrl Pts',(-7.06801146754352,1.03069226975728,13.2379912232653));
#40667=CARTESIAN_POINT('Ctrl Pts',(-7.06889154461022,-0.000133237967543647,
13.2728126690739));
#40668=CARTESIAN_POINT('Origin',(0.,0.,-2.77281266907387));
#40669=CARTESIAN_POINT('',(-7.0690926972794,-2.72305532282471E-5,9.97718733092612));
#40670=CARTESIAN_POINT('',(-7.06805535455957,-0.000126195531622297,10.2728126690739));
#40671=CARTESIAN_POINT('',(-7.0685,-3.68825033525048E-13,-2.77281266907387));
#40672=CARTESIAN_POINT('Ctrl Pts',(-7.0690926972794,-2.72305532283707E-5,
9.97718733092612));
#40673=CARTESIAN_POINT('Ctrl Pts',(-7.06909837164777,-0.0260037119360697,
9.97806489402483));
#40674=CARTESIAN_POINT('Ctrl Pts',(-7.0626311268876,-1.22423787807622,10.0185449175213));
#40675=CARTESIAN_POINT('Ctrl Pts',(-6.43419630013248,-3.58794036486512,
10.0986274014154));
#40676=CARTESIAN_POINT('Ctrl Pts',(-3.94096871160376,-6.22422394396494,
10.2174347826085));
#40677=CARTESIAN_POINT('Ctrl Pts',(-0.491681018131546,-7.35054065133146,
10.3362421638016));
#40678=CARTESIAN_POINT('Ctrl Pts',(3.07688613178757,-6.69365145660272,10.4550495449948));
#40679=CARTESIAN_POINT('Ctrl Pts',(5.8990154656956,-4.41291452737873,10.5738569261879));
#40680=CARTESIAN_POINT('Ctrl Pts',(7.2900719447016,-1.06162570218753,10.692664307381));
#40681=CARTESIAN_POINT('Ctrl Pts',(6.91259193977638,2.54720842582524,10.8114716885741));
#40682=CARTESIAN_POINT('Ctrl Pts',(4.85815028937904,5.53810200847668,10.9302790697673));
#40683=CARTESIAN_POINT('Ctrl Pts',(1.62514468290704,7.18547860967203,11.0490864509604));
#40684=CARTESIAN_POINT('Ctrl Pts',(-2.00211322794815,7.08969256829738,11.1678938321535));
#40685=CARTESIAN_POINT('Ctrl Pts',(-5.14366807368819,5.27398111849169,11.2867012133466));
#40686=CARTESIAN_POINT('Ctrl Pts',(-6.78699198309204,2.58809019405032,11.3897990462708));
#40687=CARTESIAN_POINT('Ctrl Pts',(-7.06762741654575,0.707456191694836,
11.4532944187973));
#40688=CARTESIAN_POINT('Ctrl Pts',(-7.06800228818001,-0.000105204573031432,
11.4771873309261));
#40689=CARTESIAN_POINT('Ctrl Pts',(-7.06805535455957,-0.00012619553162195,
10.2728126690739));
#40690=CARTESIAN_POINT('Ctrl Pts',(-7.06833512080673,-0.436018204661516,
10.2875321737203));
#40691=CARTESIAN_POINT('Ctrl Pts',(-6.92187198456732,-2.0444810670586,10.3418541387645));
#40692=CARTESIAN_POINT('Ctrl Pts',(-5.71614985062563,-4.64734649237981,
10.4357785642063));
#40693=CARTESIAN_POINT('Ctrl Pts',(-2.8042908954851,-6.81235283206109,10.5545859453995));
#40694=CARTESIAN_POINT('Ctrl Pts',(0.78787557894517,-7.32471505296642,10.6733933265926));
#40695=CARTESIAN_POINT('Ctrl Pts',(4.18890721731539,-6.0601365380463,10.7922007077857));
#40696=CARTESIAN_POINT('Ctrl Pts',(6.57373005855721,-3.32539796897586,10.9110080889788));
#40697=CARTESIAN_POINT('Ctrl Pts',(7.36379752129319,0.216066195757339,11.0298154701719));
#40698=CARTESIAN_POINT('Ctrl Pts',(6.36744302872343,3.70511373777206,11.1486228513651));
#40699=CARTESIAN_POINT('Ctrl Pts',(3.82637740176148,6.29531846027314,11.2674302325582));
#40700=CARTESIAN_POINT('Ctrl Pts',(0.357050971363174,7.3583091221159,11.3862376137513));
#40701=CARTESIAN_POINT('Ctrl Pts',(-3.1988943108167,6.63620928870937,11.5050449949444));
#40702=CARTESIAN_POINT('Ctrl Pts',(-5.97880318022623,4.30419691403035,11.6238523761376));
#40703=CARTESIAN_POINT('Ctrl Pts',(-6.97759561010622,1.76778178833764,11.7131082675141));
#40704=CARTESIAN_POINT('Ctrl Pts',(-7.06871225844943,0.297778996697315,
11.7627616984928));
#40705=CARTESIAN_POINT('Ctrl Pts',(-7.06841597353811,0.000180915637408539,
11.7728126690739));
#40706=CARTESIAN_POINT('Origin',(0.,0.,-2.77281266907387));
#40707=CARTESIAN_POINT('',(-7.06810297343219,0.000140531831294521,8.47718733092612));
#40708=CARTESIAN_POINT('',(-7.06910150038349,3.50688967443413E-6,8.77281266907389));
#40709=CARTESIAN_POINT('',(-7.0685,-3.68825033525048E-13,-2.77281266907387));
#40710=CARTESIAN_POINT('Ctrl Pts',(-7.06810297343219,0.000140531831294526,
8.47718733092612));
#40711=CARTESIAN_POINT('Ctrl Pts',(-7.0675551177651,-0.759365934494961,
8.50283536925235));
#40712=CARTESIAN_POINT('Ctrl Pts',(-6.75724147934998,-2.69204332921662,
8.56808586797629));
#40713=CARTESIAN_POINT('Ctrl Pts',(-5.02610585121275,-5.3861357263693,8.67293882709792));
#40714=CARTESIAN_POINT('Ctrl Pts',(-1.84527177852238,-7.1321224157929,8.79174620829105));
#40715=CARTESIAN_POINT('Ctrl Pts',(1.78321637602583,-7.14789041932932,8.91055358948417));
#40716=CARTESIAN_POINT('Ctrl Pts',(4.97910479168735,-5.42961449495844,9.02936097067729));
#40717=CARTESIAN_POINT('Ctrl Pts',(6.96708626922742,-2.39414013950925,9.14816835187041));
#40718=CARTESIAN_POINT('Ctrl Pts',(7.26488603837279,1.2221411292984,9.26697573306353));
#40719=CARTESIAN_POINT('Ctrl Pts',(5.80025930364893,4.54193682264524,9.38578311425666));
#40720=CARTESIAN_POINT('Ctrl Pts',(2.92851748521003,6.75988043010273,9.50459049544978));
#40721=CARTESIAN_POINT('Ctrl Pts',(-0.653668627291716,7.33790947178836,
9.6233978766429));
#40722=CARTESIAN_POINT('Ctrl Pts',(-4.07727786640525,6.1357968749453,9.74220525783602));
#40723=CARTESIAN_POINT('Ctrl Pts',(-6.49377691438734,3.46504353643401,9.86013507593044));
#40724=CARTESIAN_POINT('Ctrl Pts',(-7.06884230009088,1.14625680897868,9.93846243362713));
#40725=CARTESIAN_POINT('Ctrl Pts',(-7.0690926972794,-2.72305532283707E-5,
9.97718733092612));
#40726=CARTESIAN_POINT('Ctrl Pts',(-7.0691014299727,3.50647916297852E-6,
8.77281266907389));
#40727=CARTESIAN_POINT('Ctrl Pts',(-7.06906675364277,-1.16892331971989,
8.81230264894784));
#40728=CARTESIAN_POINT('Ctrl Pts',(-6.47600648320203,-3.51014035758656,
8.8913950892195));
#40729=CARTESIAN_POINT('Ctrl Pts',(-4.01809889103379,-6.17471293558617,
9.01008998988887));
#40730=CARTESIAN_POINT('Ctrl Pts',(-0.583090560721348,-7.34385484149978,
9.12889737108199));
#40731=CARTESIAN_POINT('Ctrl Pts',(2.99337274258629,-6.73141279071218,9.24770475227512));
#40732=CARTESIAN_POINT('Ctrl Pts',(5.84365817749679,-4.48596228691204,9.36651213346823));
#40733=CARTESIAN_POINT('Ctrl Pts',(7.27630017007747,-1.15223885108631,9.48531951466136));
#40734=CARTESIAN_POINT('Ctrl Pts',(6.94374664518998,2.46101220282127,9.60412689585448));
#40735=CARTESIAN_POINT('Ctrl Pts',(4.92667349274102,5.47723350159046,9.72293427704761));
#40736=CARTESIAN_POINT('Ctrl Pts',(1.71441298378659,7.16470422669678,9.84174165824072));
#40737=CARTESIAN_POINT('Ctrl Pts',(-1.91375589114147,7.11405207488272,9.96054903943386));
#40738=CARTESIAN_POINT('Ctrl Pts',(-5.07765676700238,5.33756501520463,10.079356420627));
#40739=CARTESIAN_POINT('Ctrl Pts',(-6.77036891949848,2.646732268931,10.1834442971737));
#40740=CARTESIAN_POINT('Ctrl Pts',(-7.06758241669134,0.736738382185901,
10.2479297133226));
#40741=CARTESIAN_POINT('Ctrl Pts',(-7.06805535455957,-0.00012619553162195,
10.2728126690739));
#40742=CARTESIAN_POINT('Origin',(0.,0.,-2.77281266907387));
#40743=CARTESIAN_POINT('',(-7.06834762154544,-0.000177849683210104,6.97718733092612));
#40744=CARTESIAN_POINT('',(-7.06804242201619,0.000121653731739724,7.27281266907389));
#40745=CARTESIAN_POINT('',(-7.0685,-3.68825033525048E-13,-2.77281266907387));
#40746=CARTESIAN_POINT('Ctrl Pts',(-7.06834762154545,-0.000177849683210204,
6.97718733092612));
#40747=CARTESIAN_POINT('Ctrl Pts',(-7.06865582645895,-0.320438072175684,
6.98800338408215));
#40748=CARTESIAN_POINT('Ctrl Pts',(-6.96904742463227,-1.8131255237446,7.03842189763588));
#40749=CARTESIAN_POINT('Ctrl Pts',(-5.93714558070924,-4.36147915780088,
7.12844287158734));
#40750=CARTESIAN_POINT('Ctrl Pts',(-3.13494485649586,-6.66665724611644,
7.24725025278046));
#40751=CARTESIAN_POINT('Ctrl Pts',(0.427778451839743,-7.35453626591155,
7.36605763397357));
#40752=CARTESIAN_POINT('Ctrl Pts',(3.88672475977586,-6.25824006668105,7.48486501516671));
#40753=CARTESIAN_POINT('Ctrl Pts',(6.40277028527823,-3.64372484751866,7.60367239635982));
#40754=CARTESIAN_POINT('Ctrl Pts',(7.36553445311621,-0.145259458986194,
7.72247977755295));
#40755=CARTESIAN_POINT('Ctrl Pts',(6.54145529447003,3.38844517749906,7.84128715874606));
#40756=CARTESIAN_POINT('Ctrl Pts',(4.13045046018973,6.10012926800615,7.9600945399392));
#40757=CARTESIAN_POINT('Ctrl Pts',(0.71741815768671,7.33195125989582,8.0789019211323));
#40758=CARTESIAN_POINT('Ctrl Pts',(-2.86965634847726,6.78507704688097,8.19770930232544));
#40759=CARTESIAN_POINT('Ctrl Pts',(-5.76056598999791,4.59217568972987,8.31651668351855));
#40760=CARTESIAN_POINT('Ctrl Pts',(-6.93159083568589,1.99913423513499,8.40967602638545));
#40761=CARTESIAN_POINT('Ctrl Pts',(-7.06840104726987,0.413367994389237,
8.46323290885464));
#40762=CARTESIAN_POINT('Ctrl Pts',(-7.06810297343219,0.000140531831294526,
8.47718733092612));
#40763=CARTESIAN_POINT('Ctrl Pts',(-7.06804242201619,0.000121653731739516,
7.27281266907389));
#40764=CARTESIAN_POINT('Ctrl Pts',(-7.06759172593921,-0.730084929063449,
7.29747066377764));
#40765=CARTESIAN_POINT('Ctrl Pts',(-6.77418208262749,-2.63340817566325,
7.36173111887911));
#40766=CARTESIAN_POINT('Ctrl Pts',(-5.09272545443097,-5.32318945565654,
7.46559403437827));
#40767=CARTESIAN_POINT('Ctrl Pts',(-1.9338592434572,-7.10861357519998,7.58440141557141));
#40768=CARTESIAN_POINT('Ctrl Pts',(1.69415194342111,-7.16952214081417,7.70320879676452));
#40769=CARTESIAN_POINT('Ctrl Pts',(4.91116999552812,-5.49113902665435,7.82201617795765));
#40770=CARTESIAN_POINT('Ctrl Pts',(6.93676176518449,-2.48063192515472,7.94082355915077));
#40771=CARTESIAN_POINT('Ctrl Pts',(7.27952840566287,1.13166458200723,8.0596309403439));
#40772=CARTESIAN_POINT('Ctrl Pts',(5.85631637420563,4.46942469007289,8.178438321537));
#40773=CARTESIAN_POINT('Ctrl Pts',(3.01239008261732,6.72292380777671,8.29724570273014));
#40774=CARTESIAN_POINT('Ctrl Pts',(-0.562327592835126,7.34547385900723,
8.41605308392325));
#40775=CARTESIAN_POINT('Ctrl Pts',(-4.00062729170338,6.18604718765547,8.53486046511639));
#40776=CARTESIAN_POINT('Ctrl Pts',(-6.46839400027299,3.52591514252037,8.6536678463095));
#40777=CARTESIAN_POINT('Ctrl Pts',(-7.06828828255705,1.17891875484952,8.73298524762867));
#40778=CARTESIAN_POINT('Ctrl Pts',(-7.06910152874236,0.00333299669573309,
8.77270018855014));
#40779=CARTESIAN_POINT('Ctrl Pts',(-7.0691014299727,3.50647916297852E-6,
8.77281266907389));
#40780=CARTESIAN_POINT('Origin',(0.,0.,-2.77281266907387));
#40781=CARTESIAN_POINT('',(-7.06894407494582,0.000114272372526485,5.47718733092612));
#40782=CARTESIAN_POINT('',(-7.06843645704685,-0.000181328847439488,5.77281266907388));
#40783=CARTESIAN_POINT('',(-7.0685,-3.68825033525048E-13,-2.77281266907387));
#40784=CARTESIAN_POINT('Ctrl Pts',(-7.06894407494582,0.000114272372526512,
5.47718733092612));
#40785=CARTESIAN_POINT('Ctrl Pts',(-7.06813276101183,-1.05333618941605,
5.51277385930966));
#40786=CARTESIAN_POINT('Ctrl Pts',(-6.5638901837095,-3.27986943935765,5.5879628480909));
#40787=CARTESIAN_POINT('Ctrl Pts',(-4.3160277462564,-5.97026821709139,5.70275429726988));
#40788=CARTESIAN_POINT('Ctrl Pts',(-0.942477130941647,-7.30643106777301,
5.82156167846298));
#40789=CARTESIAN_POINT('Ctrl Pts',(2.659713915357,-6.87008878974086,5.94036905965612));
#40790=CARTESIAN_POINT('Ctrl Pts',(5.61667112421129,-4.76709592654876,6.05917644084923));
#40791=CARTESIAN_POINT('Ctrl Pts',(7.21105086102525,-1.50762845892934,6.17798382204236));
#40792=CARTESIAN_POINT('Ctrl Pts',(7.05606424975171,2.11758244086091,6.29679120323547));
#40793=CARTESIAN_POINT('Ctrl Pts',(5.18931029882807,5.22907799836104,6.41559858442861));
#40794=CARTESIAN_POINT('Ctrl Pts',(2.06365456208858,7.0720243169009,6.53440596562172));
#40795=CARTESIAN_POINT('Ctrl Pts',(-1.56263387223831,7.19933146005934,6.65321334681485));
#40796=CARTESIAN_POINT('Ctrl Pts',(-4.80983482498188,5.58011532558766,6.77202072800796));
#40797=CARTESIAN_POINT('Ctrl Pts',(-6.70080011169465,2.87784082925081,6.88001205604507));
#40798=CARTESIAN_POINT('Ctrl Pts',(-7.06752734893528,0.852179387747461,
6.94840092368444));
#40799=CARTESIAN_POINT('Ctrl Pts',(-7.06834762154545,-0.000177849683210204,
6.97718733092612));
#40800=CARTESIAN_POINT('Ctrl Pts',(-7.06843645704685,-0.000181328847439211,
5.77281266907388));
#40801=CARTESIAN_POINT('Ctrl Pts',(-7.0687283062341,-0.291116138498873,
5.78263867860744));
#40802=CARTESIAN_POINT('Ctrl Pts',(-6.98006586361788,-1.7544493646656,5.83206714853871));
#40803=CARTESIAN_POINT('Ctrl Pts',(-5.9909469960723,-4.28727799719992,5.9210980788677));
#40804=CARTESIAN_POINT('Ctrl Pts',(-3.21764169554554,-6.62713968874273,
6.0399054600608));
#40805=CARTESIAN_POINT('Ctrl Pts',(0.336248045567207,-7.35928908162156,
6.15871284125395));
#40806=CARTESIAN_POINT('Ctrl Pts',(3.80856562377858,-6.30611024518239,6.27752022244705));
#40807=CARTESIAN_POINT('Ctrl Pts',(6.35694345102643,-3.72309931313607,6.39632760364018));
#40808=CARTESIAN_POINT('Ctrl Pts',(7.36315729077195,-0.236882347113499,
6.5151349848333));
#40809=CARTESIAN_POINT('Ctrl Pts',(6.58310449221504,3.30680114001436,6.63394236602642));
#40810=CARTESIAN_POINT('Ctrl Pts',(4.20602212243871,6.04827053301837,6.75274974721955));
#40811=CARTESIAN_POINT('Ctrl Pts',(0.808578961688855,7.3224585077511,6.87155712841267));
#40812=CARTESIAN_POINT('Ctrl Pts',(-2.78502157648225,6.8202531737136,6.99036450960579));
#40813=CARTESIAN_POINT('Ctrl Pts',(-5.70298923971021,4.66348713590718,7.10917189079892));
#40814=CARTESIAN_POINT('Ctrl Pts',(-6.91897017189403,2.05781460754039,7.20332127728827));
#40815=CARTESIAN_POINT('Ctrl Pts',(-7.06831557529332,0.442677804675292,
7.25786820337994));
#40816=CARTESIAN_POINT('Ctrl Pts',(-7.06804242201619,0.000121653731739516,
7.27281266907389));
#40817=CARTESIAN_POINT('Origin',(0.,0.,-2.77281266907387));
#40818=CARTESIAN_POINT('',(-7.06790662938871,2.60008083700674E-5,3.97718733092612));
#40819=CARTESIAN_POINT('',(-7.0688699538086,0.000135730005232301,4.27281266907388));
#40820=CARTESIAN_POINT('',(-7.0685,-3.68825033525048E-13,-2.77281266907387));
#40821=CARTESIAN_POINT('Ctrl Pts',(-7.06790662938871,2.60008083700913E-5,
3.97718733092612));
#40822=CARTESIAN_POINT('Ctrl Pts',(-7.06782750266918,-0.614619981437727,
3.99794187413946));
#40823=CARTESIAN_POINT('Ctrl Pts',(-6.83699561128725,-2.40215150421776,
4.05829887775052));
#40824=CARTESIAN_POINT('Ctrl Pts',(-5.34760935712609,-5.06707728913272,
4.15825834175928));
#40825=CARTESIAN_POINT('Ctrl Pts',(-2.28008659912764,-7.00524112296964,
4.2770657229524));
#40826=CARTESIAN_POINT('Ctrl Pts',(1.34057423043783,-7.24396706391966,4.39587310414552));
#40827=CARTESIAN_POINT('Ctrl Pts',(4.63601818231957,-5.72534134385619,4.51468048533865));
#40828=CARTESIAN_POINT('Ctrl Pts',(6.80678636175523,-2.81777527774835,4.63348786653177));
#40829=CARTESIAN_POINT('Ctrl Pts',(7.32626082140389,0.773369554113066,4.75229524772489));
#40830=CARTESIAN_POINT('Ctrl Pts',(6.06841954922959,4.17689864193457,4.87110262891801));
#40831=CARTESIAN_POINT('Ctrl Pts',(3.33840880410428,6.56713215545002,4.98991001011114));
#40832=CARTESIAN_POINT('Ctrl Pts',(-0.201483902833845,7.36421091002734,
5.10871739130425));
#40833=CARTESIAN_POINT('Ctrl Pts',(-3.69249758144563,6.37476742332494,5.22752477249739));
#40834=CARTESIAN_POINT('Ctrl Pts',(-6.28772905939532,3.83883593894067,5.34633215369049));
#40835=CARTESIAN_POINT('Ctrl Pts',(-7.03713150959426,1.41016055953885,5.42955300650008));
#40836=CARTESIAN_POINT('Ctrl Pts',(-7.06903563154741,0.118995928634036,
5.47317139891195));
#40837=CARTESIAN_POINT('Ctrl Pts',(-7.06894407494582,0.000114272372526512,
5.47718733092612));
#40838=CARTESIAN_POINT('Ctrl Pts',(-7.0688699538086,0.000135730005232423,
4.27281266907388));
#40839=CARTESIAN_POINT('Ctrl Pts',(-7.06797279848001,-1.02403807532536,
4.30740915383496));
#40840=CARTESIAN_POINT('Ctrl Pts',(-6.58508986586626,-3.22139801692903,
4.38160809899374));
#40841=CARTESIAN_POINT('Ctrl Pts',(-4.38996945438879,-5.91611077690027,
4.49540950455022));
#40842=CARTESIAN_POINT('Ctrl Pts',(-1.03330302320227,-7.29414034669358,
4.61421688574334));
#40843=CARTESIAN_POINT('Ctrl Pts',(2.57403776474647,-6.90264645774946,4.73302426693647));
#40844=CARTESIAN_POINT('Ctrl Pts',(5.5569293384078,-4.83660364956287,4.85183164812959));
#40845=CARTESIAN_POINT('Ctrl Pts',(7.19173651068846,-1.59722399676838,4.97063902932272));
#40846=CARTESIAN_POINT('Ctrl Pts',(7.08186290362403,2.02963453589456,5.08944641051583));
#40847=CARTESIAN_POINT('Ctrl Pts',(5.25396332723401,5.16411346613359,5.20825379170895));
#40848=CARTESIAN_POINT('Ctrl Pts',(2.15147745047193,7.04580324130137,5.32706117290208));
#40849=CARTESIAN_POINT('Ctrl Pts',(-1.47294653532043,7.21821494824792,5.4458685540952));
#40850=CARTESIAN_POINT('Ctrl Pts',(-4.74004075724321,5.63952233391227,5.56467593528832));
#40851=CARTESIAN_POINT('Ctrl Pts',(-6.68212139988246,2.9364259970353,5.67365730694789));
#40852=CARTESIAN_POINT('Ctrl Pts',(-7.06755204583654,0.881458978407337,
5.74303621820974));
#40853=CARTESIAN_POINT('Ctrl Pts',(-7.06843645704685,-0.000181328847439211,
5.77281266907388));
#40854=CARTESIAN_POINT('Origin',(0.,0.,-2.77281266907387));
#40855=CARTESIAN_POINT('',(-7.06879387608848,-0.000152214530812696,2.47718733092612));
#40856=CARTESIAN_POINT('',(-7.06790105247164,-1.00512679984677E-6,2.77281266907389));
#40857=CARTESIAN_POINT('',(-7.0685,-3.68825033525048E-13,-2.77281266907387));
#40858=CARTESIAN_POINT('Ctrl Pts',(-7.06879387608848,-0.000152214530812871,
2.47718733092612));
#40859=CARTESIAN_POINT('Ctrl Pts',(-7.06896001159515,-0.175485562544569,
2.48310988896927));
#40860=CARTESIAN_POINT('Ctrl Pts',(-7.0198256726627,-1.52313020894557,2.52863490741013));
#40861=CARTESIAN_POINT('Ctrl Pts',(-6.19395711760227,-3.9883697563648,2.61376238624869));
#40862=CARTESIAN_POINT('Ctrl Pts',(-3.53871699613534,-6.46139923806788,
2.73256976744181));
#40863=CARTESIAN_POINT('Ctrl Pts',(-0.0250011063573954,-7.36692425873726,
2.85137714863493));
#40864=CARTESIAN_POINT('Ctrl Pts',(3.49477993190855,-6.48526879308302,2.97018452982806));
#40865=CARTESIAN_POINT('Ctrl Pts',(6.16674412284828,-4.03031822733696,3.08899191102118));
#40866=CARTESIAN_POINT('Ctrl Pts',(7.34268577093533,-0.597631792820449,
3.2077992922143));
#40867=CARTESIAN_POINT('Ctrl Pts',(6.73732707323029,2.98003724789039,3.32660667340742));
#40868=CARTESIAN_POINT('Ctrl Pts',(4.4975251459451,5.83476354722511,3.44541405460054));
#40869=CARTESIAN_POINT('Ctrl Pts',(1.16664519249845,7.27400419887887,3.56422143579367));
#40870=CARTESIAN_POINT('Ctrl Pts',(-2.44725728835037,6.94860632465767,3.68302881698679));
#40871=CARTESIAN_POINT('Ctrl Pts',(-5.46746689033045,4.93750988795068,3.80183619817991));
#40872=CARTESIAN_POINT('Ctrl Pts',(-6.86539920913079,2.28916439736259,3.89988903615969));
#40873=CARTESIAN_POINT('Ctrl Pts',(-7.06797848709435,0.558207236212538,
3.95833941374176));
#40874=CARTESIAN_POINT('Ctrl Pts',(-7.06790662938871,2.60008083700913E-5,
3.97718733092612));
#40875=CARTESIAN_POINT('Ctrl Pts',(-7.06790105247164,-1.00512680008963E-6,
2.77281266907389));
#40876=CARTESIAN_POINT('Ctrl Pts',(-7.06790396260581,-0.585328167239678,
2.79257716866476));
#40877=CARTESIAN_POINT('Ctrl Pts',(-6.8519294853734,-2.34348310332654,2.85194412865334));
#40878=CARTESIAN_POINT('Ctrl Pts',(-5.41023469503032,-5.0001559055375,2.95091354903963));
#40879=CARTESIAN_POINT('Ctrl Pts',(-2.36706189309541,-6.97633259881565,
3.06972093023276));
#40880=CARTESIAN_POINT('Ctrl Pts',(1.25034876951077,-7.26008446848898,3.18852831142588));
#40881=CARTESIAN_POINT('Ctrl Pts',(4.56443081844987,-5.78257467211716,3.307335692619));
#40882=CARTESIAN_POINT('Ctrl Pts',(6.7712038460194,-2.90223999880672,3.42614307381212));
#40883=CARTESIAN_POINT('Ctrl Pts',(7.33531530143303,0.682164176415201,3.54495045500525));
#40884=CARTESIAN_POINT('Ctrl Pts',(6.11991445160226,4.10107859472268,3.66375783619837));
#40885=CARTESIAN_POINT('Ctrl Pts',(3.41985171252147,6.5250910184752,3.78256521739149));
#40886=CARTESIAN_POINT('Ctrl Pts',(-0.109850647279407,7.36614766145199,
3.90137259858461));
#40887=CARTESIAN_POINT('Ctrl Pts',(-3.61290376699451,6.42021221654385,4.02017997977773));
#40888=CARTESIAN_POINT('Ctrl Pts',(-6.2394837636286,3.91676408511378,4.13898736097086));
#40889=CARTESIAN_POINT('Ctrl Pts',(-7.02831730228861,1.46882013834326,4.2231982574029));
#40890=CARTESIAN_POINT('Ctrl Pts',(-7.06899976866546,0.148329662208865,
4.26780669343725));
#40891=CARTESIAN_POINT('Ctrl Pts',(-7.0688699538086,0.000135730005232423,
4.27281266907388));
#40892=CARTESIAN_POINT('Origin',(0.,0.,-2.77281266907387));
#40893=CARTESIAN_POINT('',(-7.0685211611855,0.000181853424906659,0.977187330926116));
#40894=CARTESIAN_POINT('',(-7.06887577069393,-0.000134259091651989,1.27281266907389));
#40895=CARTESIAN_POINT('',(-7.0685,-3.68825033525048E-13,-2.77281266907387));
#40896=CARTESIAN_POINT('Ctrl Pts',(-7.06852116118549,0.000181853424906647,
0.977187330926117));
#40897=CARTESIAN_POINT('Ctrl Pts',(-7.06759165261753,-0.908565991214031,
1.00788036419678));
#40898=CARTESIAN_POINT('Ctrl Pts',(-6.66445125668807,-2.9906520072978,1.07817585786515));
#40899=CARTESIAN_POINT('Ctrl Pts',(-4.67477113205871,-5.69374237749066,
1.18807381193122));
#40900=CARTESIAN_POINT('Ctrl Pts',(-1.38971041869972,-7.23470180222814,
1.30688119312434));
#40901=CARTESIAN_POINT('Ctrl Pts',(2.23248728958399,-7.02055517652312,1.42568857431747));
#40902=CARTESIAN_POINT('Ctrl Pts',(5.31309433455675,-5.10325661323295,1.54449595551059));
#40903=CARTESIAN_POINT('Ctrl Pts',(7.10477015790912,-1.94793192835274,1.66330333670371));
#40904=CARTESIAN_POINT('Ctrl Pts',(7.17286283343114,1.67995141886001,1.78211071789683));
#40905=CARTESIAN_POINT('Ctrl Pts',(5.50085338730159,4.90028675314958,1.90091809908995));
#40906=CARTESIAN_POINT('Ctrl Pts',(2.49436329953803,6.93183595449864,2.01972548028308));
#40907=CARTESIAN_POINT('Ctrl Pts',(-1.1172473609771,7.28175504193768,2.1385328614762));
#40908=CARTESIAN_POINT('Ctrl Pts',(-4.45781917027722,5.86515526715037,2.25734024266932));
#40909=CARTESIAN_POINT('Ctrl Pts',(-6.60432779697333,3.16724420624364,2.37022506581929));
#40910=CARTESIAN_POINT('Ctrl Pts',(-7.06784911073517,0.99691864532032,2.44350742857156));
#40911=CARTESIAN_POINT('Ctrl Pts',(-7.06879387608848,-0.000152214530812871,
2.47718733092612));
#40912=CARTESIAN_POINT('Ctrl Pts',(-7.06887577069393,-0.000134259091651625,
1.27281266907389));
#40913=CARTESIAN_POINT('Ctrl Pts',(-7.06900268511687,-0.146153139652322,
1.27774518349456));
#40914=CARTESIAN_POINT('Ctrl Pts',(-7.02898406704184,-1.46446746156119,
1.32228015831295));
#40915=CARTESIAN_POINT('Ctrl Pts',(-6.24309683168348,-3.91100251149225,
1.40641759352904));
#40916=CARTESIAN_POINT('Ctrl Pts',(-3.61882898585832,-6.41687425365725,
1.52522497472216));
#40917=CARTESIAN_POINT('Ctrl Pts',(-0.116650592004996,-7.36604311957603,
1.64403235591529));
#40918=CARTESIAN_POINT('Ctrl Pts',(3.41382667831815,-6.5282452403422,1.76283973710841));
#40919=CARTESIAN_POINT('Ctrl Pts',(6.11612597108606,-4.10672639074461,1.88164711830153));
#40920=CARTESIAN_POINT('Ctrl Pts',(7.33468244243266,-0.688935413517191,
2.00045449949465));
#40921=CARTESIAN_POINT('Ctrl Pts',(6.77388013677175,2.89598798778839,2.11926188068778));
#40922=CARTESIAN_POINT('Ctrl Pts',(4.56976700382019,5.77835859632846,2.2380692618809));
#40923=CARTESIAN_POINT('Ctrl Pts',(1.25705031644168,7.25892712704843,2.35687664307402));
#40924=CARTESIAN_POINT('Ctrl Pts',(-2.36062074769956,6.97851475753138,2.47568402426714));
#40925=CARTESIAN_POINT('Ctrl Pts',(-5.40561654216747,5.00514818301045,2.59449140546027));
#40926=CARTESIAN_POINT('Ctrl Pts',(-6.85083513592755,2.34783644208199,2.69353428706251));
#40927=CARTESIAN_POINT('Ctrl Pts',(-7.06789813152101,0.587501716496959,
2.75297470826705));
#40928=CARTESIAN_POINT('Ctrl Pts',(-7.06790105247164,-1.00512680008963E-6,
2.77281266907389));
#40929=CARTESIAN_POINT('Ctrl Pts',(-3.08141029750819,6.36149375763354,-0.494500505560914));
#40930=CARTESIAN_POINT('Ctrl Pts',(-4.13669558412972,5.85032970200549,-0.454898045163206));
#40931=CARTESIAN_POINT('Ctrl Pts',(-5.98693791583793,4.29325218121263,-0.375693124367791));
#40932=CARTESIAN_POINT('Ctrl Pts',(-7.31006311005933,0.913880564558005,
-0.25688574317467));
#40933=CARTESIAN_POINT('Ctrl Pts',(-6.85969295893001,-2.68627098725521,
-0.138078361981547));
#40934=CARTESIAN_POINT('Ctrl Pts',(-4.74525181548372,-5.63519834469009,
-0.0192709807884249));
#40935=CARTESIAN_POINT('Ctrl Pts',(-1.47960575920872,-7.21682451563664,
0.0995364004046977));
#40936=CARTESIAN_POINT('Ctrl Pts',(2.14497044005655,-7.04780045183455,0.21834378159782));
#40937=CARTESIAN_POINT('Ctrl Pts',(5.24919481691,-5.16895421862038,0.337151162790942));
#40938=CARTESIAN_POINT('Ctrl Pts',(7.07998577213964,-2.03617489938541,0.455958543984065));
#40939=CARTESIAN_POINT('Ctrl Pts',(7.19320815162393,1.59058620557498,0.574765925177186));
#40940=CARTESIAN_POINT('Ctrl Pts',(5.56139171256912,4.83147080423204,0.693573306370309));
#40941=CARTESIAN_POINT('Ctrl Pts',(2.5804088453257,6.9002678057359,0.812380687563431));
#40942=CARTESIAN_POINT('Ctrl Pts',(-1.02656909712053,7.29509087359264,0.931188068756555));
#40943=CARTESIAN_POINT('Ctrl Pts',(-4.3845061645243,5.92016094290675,1.04999544994967));
#40944=CARTESIAN_POINT('Ctrl Pts',(-6.67878313815982,3.10902782828873,1.1688028311428));
#40945=CARTESIAN_POINT('Ctrl Pts',(-7.35281932448621,-0.456340249290331,
1.28761021233592));
#40946=CARTESIAN_POINT('Ctrl Pts',(-6.24309683168348,-3.91100251149225,
1.40641759352904));
#40947=CARTESIAN_POINT('Ctrl Pts',(-3.61882898585832,-6.41687425365725,
1.52522497472216));
#40948=CARTESIAN_POINT('Ctrl Pts',(-0.116650592004996,-7.36604311957603,
1.64403235591529));
#40949=CARTESIAN_POINT('Ctrl Pts',(3.41382667831815,-6.5282452403422,1.76283973710841));
#40950=CARTESIAN_POINT('Ctrl Pts',(6.11612597108606,-4.10672639074461,1.88164711830153));
#40951=CARTESIAN_POINT('Ctrl Pts',(7.33468244243266,-0.688935413517191,
2.00045449949465));
#40952=CARTESIAN_POINT('Ctrl Pts',(6.77388013677175,2.89598798778839,2.11926188068778));
#40953=CARTESIAN_POINT('Ctrl Pts',(4.56976700382019,5.77835859632846,2.2380692618809));
#40954=CARTESIAN_POINT('Ctrl Pts',(1.25705031644168,7.25892712704843,2.35687664307402));
#40955=CARTESIAN_POINT('Ctrl Pts',(-2.36062074769956,6.97851475753138,2.47568402426714));
#40956=CARTESIAN_POINT('Ctrl Pts',(-5.40561654216747,5.00514818301045,2.59449140546027));
#40957=CARTESIAN_POINT('Ctrl Pts',(-7.13923569377689,1.81755666864683,2.71329878665339));
#40958=CARTESIAN_POINT('Ctrl Pts',(-7.14091051238772,-1.81096537490967,
2.83210616784651));
#40959=CARTESIAN_POINT('Ctrl Pts',(-5.41023469503032,-5.0001559055375,2.95091354903963));
#40960=CARTESIAN_POINT('Ctrl Pts',(-2.36706189309541,-6.97633259881565,
3.06972093023276));
#40961=CARTESIAN_POINT('Ctrl Pts',(1.25034876951077,-7.26008446848898,3.18852831142588));
#40962=CARTESIAN_POINT('Ctrl Pts',(4.56443081844987,-5.78257467211716,3.307335692619));
#40963=CARTESIAN_POINT('Ctrl Pts',(6.7712038460194,-2.90223999880672,3.42614307381212));
#40964=CARTESIAN_POINT('Ctrl Pts',(7.33531530143303,0.682164176415201,3.54495045500525));
#40965=CARTESIAN_POINT('Ctrl Pts',(6.11991445160226,4.10107859472268,3.66375783619837));
#40966=CARTESIAN_POINT('Ctrl Pts',(3.41985171252147,6.5250910184752,3.78256521739149));
#40967=CARTESIAN_POINT('Ctrl Pts',(-0.109850647279407,7.36614766145199,
3.90137259858461));
#40968=CARTESIAN_POINT('Ctrl Pts',(-3.61290376699451,6.42021221654385,4.02017997977773));
#40969=CARTESIAN_POINT('Ctrl Pts',(-6.2394837636286,3.91676408511378,4.13898736097086));
#40970=CARTESIAN_POINT('Ctrl Pts',(-7.35239492947897,0.463127775019019,
4.25779474216397));
#40971=CARTESIAN_POINT('Ctrl Pts',(-6.68165035425043,-3.10286111171082,
4.3766021233571));
#40972=CARTESIAN_POINT('Ctrl Pts',(-4.38996945438879,-5.91611077690027,
4.49540950455022));
#40973=CARTESIAN_POINT('Ctrl Pts',(-1.03330302320227,-7.29414034669358,
4.61421688574334));
#40974=CARTESIAN_POINT('Ctrl Pts',(2.57403776474647,-6.90264645774946,4.73302426693647));
#40975=CARTESIAN_POINT('Ctrl Pts',(5.5569293384078,-4.83660364956287,4.85183164812959));
#40976=CARTESIAN_POINT('Ctrl Pts',(7.19173651068846,-1.59722399676838,4.97063902932272));
#40977=CARTESIAN_POINT('Ctrl Pts',(7.08186290362403,2.02963453589456,5.08944641051583));
#40978=CARTESIAN_POINT('Ctrl Pts',(5.25396332723401,5.16411346613359,5.20825379170895));
#40979=CARTESIAN_POINT('Ctrl Pts',(2.15147745047193,7.04580324130137,5.32706117290208));
#40980=CARTESIAN_POINT('Ctrl Pts',(-1.47294653532043,7.21821494824792,5.4458685540952));
#40981=CARTESIAN_POINT('Ctrl Pts',(-4.74004075724321,5.63952233391227,5.56467593528832));
#40982=CARTESIAN_POINT('Ctrl Pts',(-6.85722382903087,2.69270865367817,5.68348331648145));
#40983=CARTESIAN_POINT('Ctrl Pts',(-7.31087729341474,-0.907343229244046,
5.80229069767456));
#40984=CARTESIAN_POINT('Ctrl Pts',(-5.9909469960723,-4.28727799719992,5.9210980788677));
#40985=CARTESIAN_POINT('Ctrl Pts',(-3.21764169554554,-6.62713968874273,
6.0399054600608));
#40986=CARTESIAN_POINT('Ctrl Pts',(0.336248045567207,-7.35928908162156,
6.15871284125395));
#40987=CARTESIAN_POINT('Ctrl Pts',(3.80856562377858,-6.30611024518239,6.27752022244705));
#40988=CARTESIAN_POINT('Ctrl Pts',(6.35694345102643,-3.72309931313607,6.39632760364018));
#40989=CARTESIAN_POINT('Ctrl Pts',(7.36315729077195,-0.236882347113499,
6.5151349848333));
#40990=CARTESIAN_POINT('Ctrl Pts',(6.58310449221504,3.30680114001436,6.63394236602642));
#40991=CARTESIAN_POINT('Ctrl Pts',(4.20602212243871,6.04827053301837,6.75274974721955));
#40992=CARTESIAN_POINT('Ctrl Pts',(0.808578961688855,7.3224585077511,6.87155712841267));
#40993=CARTESIAN_POINT('Ctrl Pts',(-2.78502157648225,6.8202531737136,6.99036450960579));
#40994=CARTESIAN_POINT('Ctrl Pts',(-5.70298923971021,4.66348713590718,7.10917189079892));
#40995=CARTESIAN_POINT('Ctrl Pts',(-7.23743907013845,1.37538148928055,7.22797927199203));
#40996=CARTESIAN_POINT('Ctrl Pts',(-7.01612089953035,-2.24638510905758,
7.34678665318516));
#40997=CARTESIAN_POINT('Ctrl Pts',(-5.09272545443097,-5.32318945565654,
7.46559403437827));
#40998=CARTESIAN_POINT('Ctrl Pts',(-1.9338592434572,-7.10861357519998,7.58440141557141));
#40999=CARTESIAN_POINT('Ctrl Pts',(1.69415194342111,-7.16952214081417,7.70320879676452));
#41000=CARTESIAN_POINT('Ctrl Pts',(4.91116999552812,-5.49113902665435,7.82201617795765));
#41001=CARTESIAN_POINT('Ctrl Pts',(6.93676176518449,-2.48063192515472,7.94082355915077));
#41002=CARTESIAN_POINT('Ctrl Pts',(7.27952840566287,1.13166458200723,8.0596309403439));
#41003=CARTESIAN_POINT('Ctrl Pts',(5.85631637420563,4.46942469007289,8.178438321537));
#41004=CARTESIAN_POINT('Ctrl Pts',(3.01239008261732,6.72292380777671,8.29724570273014));
#41005=CARTESIAN_POINT('Ctrl Pts',(-0.562327592835126,7.34547385900723,
8.41605308392325));
#41006=CARTESIAN_POINT('Ctrl Pts',(-4.00062729170338,6.18604718765547,8.53486046511639));
#41007=CARTESIAN_POINT('Ctrl Pts',(-6.46839400027299,3.52591514252037,8.6536678463095));
#41008=CARTESIAN_POINT('Ctrl Pts',(-7.36695935271188,0.0104129973246502,
8.77247522750263));
#41009=CARTESIAN_POINT('Ctrl Pts',(-6.47833570485983,-3.50761529107176,
8.89128260869574));
#41010=CARTESIAN_POINT('Ctrl Pts',(-4.01809889103379,-6.17471293558617,
9.01008998988887));
#41011=CARTESIAN_POINT('Ctrl Pts',(-0.583090560721348,-7.34385484149978,
9.12889737108199));
#41012=CARTESIAN_POINT('Ctrl Pts',(2.99337274258629,-6.73141279071218,9.24770475227512));
#41013=CARTESIAN_POINT('Ctrl Pts',(5.84365817749679,-4.48596228691204,9.36651213346823));
#41014=CARTESIAN_POINT('Ctrl Pts',(7.27630017007747,-1.15223885108631,9.48531951466136));
#41015=CARTESIAN_POINT('Ctrl Pts',(6.94374664518998,2.46101220282127,9.60412689585448));
#41016=CARTESIAN_POINT('Ctrl Pts',(4.92667349274102,5.47723350159046,9.72293427704761));
#41017=CARTESIAN_POINT('Ctrl Pts',(1.71441298378659,7.16470422669678,9.84174165824072));
#41018=CARTESIAN_POINT('Ctrl Pts',(-1.91375589114147,7.11405207488272,9.96054903943386));
#41019=CARTESIAN_POINT('Ctrl Pts',(-5.07765676700238,5.33756501520463,10.079356420627));
#41020=CARTESIAN_POINT('Ctrl Pts',(-7.00974246827655,2.26621028668262,10.1981638018201));
#41021=CARTESIAN_POINT('Ctrl Pts',(-7.24129827188348,-1.35491618657003,
10.3169711830132));
#41022=CARTESIAN_POINT('Ctrl Pts',(-5.71614985062563,-4.64734649237981,
10.4357785642063));
#41023=CARTESIAN_POINT('Ctrl Pts',(-2.8042908954851,-6.81235283206109,10.5545859453995));
#41024=CARTESIAN_POINT('Ctrl Pts',(0.78787557894517,-7.32471505296642,10.6733933265926));
#41025=CARTESIAN_POINT('Ctrl Pts',(4.18890721731539,-6.0601365380463,10.7922007077857));
#41026=CARTESIAN_POINT('Ctrl Pts',(6.57373005855721,-3.32539796897586,10.9110080889788));
#41027=CARTESIAN_POINT('Ctrl Pts',(7.36379752129319,0.216066195757339,11.0298154701719));
#41028=CARTESIAN_POINT('Ctrl Pts',(6.36744302872343,3.70511373777206,11.1486228513651));
#41029=CARTESIAN_POINT('Ctrl Pts',(3.82637740176148,6.29531846027314,11.2674302325582));
#41030=CARTESIAN_POINT('Ctrl Pts',(0.357050971363174,7.3583091221159,11.3862376137513));
#41031=CARTESIAN_POINT('Ctrl Pts',(-3.1988943108167,6.63620928870937,11.5050449949444));
#41032=CARTESIAN_POINT('Ctrl Pts',(-5.97880318022623,4.30419691403035,11.6238523761376));
#41033=CARTESIAN_POINT('Ctrl Pts',(-7.30828307359288,0.928007017151897,
11.7426597573307));
#41034=CARTESIAN_POINT('Ctrl Pts',(-6.86480855900118,-2.67331293498022,
11.8614671385238));
#41035=CARTESIAN_POINT('Ctrl Pts',(-4.75596440127724,-5.62609998399613,
11.9802745197169));
#41036=CARTESIAN_POINT('Ctrl Pts',(-1.49334612632416,-7.21402218195007,
12.09908190091));
#41037=CARTESIAN_POINT('Ctrl Pts',(2.13155081922184,-7.05185717004641,12.2178892821032));
#41038=CARTESIAN_POINT('Ctrl Pts',(5.23934363589174,-5.17894550161347,12.3366966632963));
#41039=CARTESIAN_POINT('Ctrl Pts',(7.07609706408506,-2.04964636860042,12.4555040444894));
#41040=CARTESIAN_POINT('Ctrl Pts',(7.19622280814078,1.5768868890101,12.5743114256825));
#41041=CARTESIAN_POINT('Ctrl Pts',(5.57058035869953,4.82087544613853,12.6931188068757));
#41042=CARTESIAN_POINT('Ctrl Pts',(2.5935399939851,6.89534177632834,12.8119261880688));
#41043=CARTESIAN_POINT('Ctrl Pts',(-1.01267712366536,7.29703316651084,12.9307335692619));
#41044=CARTESIAN_POINT('Ctrl Pts',(-4.37323069894997,5.92849559402285,13.049540950455));
#41045=CARTESIAN_POINT('Ctrl Pts',(-6.67284563268825,3.12174071671263,13.1683483316481));
#41046=CARTESIAN_POINT('Ctrl Pts',(-7.3536873644992,-0.442347762287138,
13.2871557128413));
#41047=CARTESIAN_POINT('Ctrl Pts',(-6.25050664162124,-3.89909682044781,
13.4059630940344));
#41048=CARTESIAN_POINT('Ctrl Pts',(-3.63108720070629,-6.40999851148318,
13.5247704752275));
#41049=CARTESIAN_POINT('Ctrl Pts',(-0.130578947762305,-7.3657578324409,
13.6435778564207));
#41050=CARTESIAN_POINT('Ctrl Pts',(3.40120320632095,-6.5348310696329,13.7623852376137));
#41051=CARTESIAN_POINT('Ctrl Pts',(6.10869718244117,-4.11816204547854,13.8811926188069));
#41052=CARTESIAN_POINT('Ctrl Pts',(6.9243752846715,-1.84163918696265,13.9603975396023));
#41053=CARTESIAN_POINT('Ctrl Pts',(7.03625248964568,-0.674420604634066,
14.));
#41054=CARTESIAN_POINT('Ctrl Pts',(-3.20586989147275,6.61843744693175,-0.329667003707276));
#41055=CARTESIAN_POINT('Ctrl Pts',(-4.30377864125201,6.08662723753957,-0.290064543309568));
#41056=CARTESIAN_POINT('Ctrl Pts',(-6.22875312061569,4.46665863204891,-0.210859622514153));
#41057=CARTESIAN_POINT('Ctrl Pts',(-7.60531995633817,0.950792625275473,
-0.0920522413210315));
#41058=CARTESIAN_POINT('Ctrl Pts',(-7.13675914550065,-2.79477072084242,
0.0267551398720911));
#41059=CARTESIAN_POINT('Ctrl Pts',(-4.93691474160959,-5.86280662472249,
0.145562521065213));
#41060=CARTESIAN_POINT('Ctrl Pts',(-1.53936772345208,-7.50831541175523,
0.264369902258336));
#41061=CARTESIAN_POINT('Ctrl Pts',(2.23160679297952,-7.33246438746429,0.383177283451458));
#41062=CARTESIAN_POINT('Ctrl Pts',(5.46121223506488,-5.37773068171951,0.50198466464458));
#41063=CARTESIAN_POINT('Ctrl Pts',(7.36594968781422,-2.11841694985929,0.620792045837702));
#41064=CARTESIAN_POINT('Ctrl Pts',(7.48374517182464,1.65483072162386,0.739599427030824));
#41065=CARTESIAN_POINT('Ctrl Pts',(5.78601890842942,5.02661615538266,0.858406808223948));
#41066=CARTESIAN_POINT('Ctrl Pts',(2.68463275780226,7.17897282922568,0.977214189417068));
#41067=CARTESIAN_POINT('Ctrl Pts',(-1.0680327000388,7.58974298428242,1.09602157061019));
#41068=CARTESIAN_POINT('Ctrl Pts',(-4.56159840615571,6.15927899471405,1.21482895180331));
#41069=CARTESIAN_POINT('Ctrl Pts',(-6.94854229299388,3.23460290715646,1.33363633299644));
#41070=CARTESIAN_POINT('Ctrl Pts',(-7.64980311413618,-0.474772044037771,
1.45244371418956));
#41071=CARTESIAN_POINT('Ctrl Pts',(-6.49525841411903,-4.06896972052259,
1.57125109538268));
#41072=CARTESIAN_POINT('Ctrl Pts',(-3.76499517040421,-6.67605478692726,
1.6900584765758));
#41073=CARTESIAN_POINT('Ctrl Pts',(-0.121362163628049,-7.66356102445527,
1.80886585776892));
#41074=CARTESIAN_POINT('Ctrl Pts',(3.55171272439013,-6.79192409952275,1.92767323896205));
#41075=CARTESIAN_POINT('Ctrl Pts',(6.36315914145388,-4.27259897821829,2.04648062015517));
#41076=CARTESIAN_POINT('Ctrl Pts',(7.63093367498759,-0.716761835043583,
2.16528800134829));
#41077=CARTESIAN_POINT('Ctrl Pts',(7.04748030357494,3.0129582884906,2.28409538254141));
#41078=CARTESIAN_POINT('Ctrl Pts',(4.75434201684852,6.01174918545651,2.40290276373454));
#41079=CARTESIAN_POINT('Ctrl Pts',(1.30782316292173,7.55211856720863,2.52171014492766));
#41080=CARTESIAN_POINT('Ctrl Pts',(-2.45596731676912,7.26038021176852,2.64051752612078));
#41081=CARTESIAN_POINT('Ctrl Pts',(-5.6239519065006,5.20730844420442,2.7593249073139));
#41082=CARTESIAN_POINT('Ctrl Pts',(-7.4275927413221,1.89096862718099,2.87813228850702));
#41083=CARTESIAN_POINT('Ctrl Pts',(-7.42933520663497,-1.88411110802654,
2.99693966970015));
#41084=CARTESIAN_POINT('Ctrl Pts',(-5.62875658870384,-5.20211452632421,
3.11574705089327));
#41085=CARTESIAN_POINT('Ctrl Pts',(-2.46266862302097,-7.25810991464812,
3.2345544320864));
#41086=CARTESIAN_POINT('Ctrl Pts',(1.30085093739578,-7.55332265420782,3.35336181327951));
#41087=CARTESIAN_POINT('Ctrl Pts',(4.74879030047114,-6.01613555050572,3.47216919447264));
#41088=CARTESIAN_POINT('Ctrl Pts',(7.04469591619532,-3.01946282113952,3.59097657566576));
#41089=CARTESIAN_POINT('Ctrl Pts',(7.6315920954571,0.709717104528156,3.70978395685888));
#41090=CARTESIAN_POINT('Ctrl Pts',(6.3671006404588,4.26672306509026,3.82859133805201));
#41091=CARTESIAN_POINT('Ctrl Pts',(3.55798111252501,6.78864247716865,3.94739871924512));
#41092=CARTESIAN_POINT('Ctrl Pts',(-0.114287565974772,7.66366978882619,
4.06620610043825));
#41093=CARTESIAN_POINT('Ctrl Pts',(-3.75883062919679,6.67952757168615,4.18501348163137));
#41094=CARTESIAN_POINT('Ctrl Pts',(-6.49149941256627,4.07496400678033,4.30382086282449));
#41095=CARTESIAN_POINT('Ctrl Pts',(-7.64936157761737,0.481833721085094,
4.42262824401762));
#41096=CARTESIAN_POINT('Ctrl Pts',(-6.95152531727491,-3.22818711403002,
4.54143562521074));
#41097=CARTESIAN_POINT('Ctrl Pts',(-4.56728236083685,-6.15506524062029,
4.66024300640386));
#41098=CARTESIAN_POINT('Ctrl Pts',(-1.07503861252453,-7.58875406516016,
4.77905038759698));
#41099=CARTESIAN_POINT('Ctrl Pts',(2.67800434631753,-7.18144755609954,4.8978577687901));
#41100=CARTESIAN_POINT('Ctrl Pts',(5.78137629690187,-5.03195631872185,5.01666514998322));
#41101=CARTESIAN_POINT('Ctrl Pts',(7.48221409062784,-1.66173661628843,5.13547253117636));
#41102=CARTESIAN_POINT('Ctrl Pts',(7.36790263751166,2.11161241804746,5.25427991236947));
#41103=CARTESIAN_POINT('Ctrl Pts',(5.466173347737,5.37269440899007,5.3730872935626));
#41104=CARTESIAN_POINT('Ctrl Pts',(2.23837662456966,7.33038650866949,5.49189467475571));
#41105=CARTESIAN_POINT('Ctrl Pts',(-1.53243953041611,7.50976200458587,5.61070205594885));
#41106=CARTESIAN_POINT('Ctrl Pts',(-4.93149320630494,5.86730526187889,5.72950943714195));
#41107=CARTESIAN_POINT('Ctrl Pts',(-7.13419028629737,2.80146840760407,5.84831681833509));
#41108=CARTESIAN_POINT('Ctrl Pts',(-7.60616702493768,-0.943991243950004,
5.9671241995282));
#41109=CARTESIAN_POINT('Ctrl Pts',(-6.23292412946393,-4.46044314796747,
6.08593158072133));
#41110=CARTESIAN_POINT('Ctrl Pts',(-3.34760373898875,-6.89481294065417,
6.20473896191445));
#41111=CARTESIAN_POINT('Ctrl Pts',(0.349829260394867,-7.65653418776898,
6.32354634310758));
#41112=CARTESIAN_POINT('Ctrl Pts',(3.96239535930786,-6.56081696867387,6.44235372430069));
#41113=CARTESIAN_POINT('Ctrl Pts',(6.61370335132607,-3.8734770246591,6.56116110549382));
#41114=CARTESIAN_POINT('Ctrl Pts',(7.66055863568464,-0.246450135201629,
6.67996848668693));
#41115=CARTESIAN_POINT('Ctrl Pts',(6.84899914207391,3.44036437485541,6.79877586788007));
#41116=CARTESIAN_POINT('Ctrl Pts',(4.375905310662,6.29256299070766,6.91758324907318));
#41117=CARTESIAN_POINT('Ctrl Pts',(0.841237841728794,7.6182160099033,7.03639063026631));
#41118=CARTESIAN_POINT('Ctrl Pts',(-2.8975098922615,7.0957263690302,7.15519801145942));
#41119=CARTESIAN_POINT('Ctrl Pts',(-5.93333562549746,4.85184754862579,7.27400539265256));
#41120=CARTESIAN_POINT('Ctrl Pts',(-7.52976259769374,1.43093378682455,7.39281277384567));
#41121=CARTESIAN_POINT('Ctrl Pts',(-7.29950528331981,-2.33711764759276,
7.5116201550388));
#41122=CARTESIAN_POINT('Ctrl Pts',(-5.2984230023181,-5.5381955516585,7.63042753623192));
#41123=CARTESIAN_POINT('Ctrl Pts',(-2.01196871703817,-7.3957337811446,7.74923491742504));
#41124=CARTESIAN_POINT('Ctrl Pts',(1.76257952775252,-7.45910247203048,7.86804229861817));
#41125=CARTESIAN_POINT('Ctrl Pts',(5.10953443405443,-5.71292868388146,7.98684967981128));
#41126=CARTESIAN_POINT('Ctrl Pts',(7.21694079665652,-2.58082580145546,8.10565706100442));
#41127=CARTESIAN_POINT('Ctrl Pts',(7.5735519410405,1.17737304040193,8.22446444219752));
#41128=CARTESIAN_POINT('Ctrl Pts',(6.0928557142121,4.64994683041607,8.34327182339065));
#41129=CARTESIAN_POINT('Ctrl Pts',(3.13406191802616,6.99446582477044,8.46207920458377));
#41130=CARTESIAN_POINT('Ctrl Pts',(-0.585040265644679,7.64216096189278,
8.58088658577689));
#41131=CARTESIAN_POINT('Ctrl Pts',(-4.16221448725848,6.43590450845561,8.69969396697002));
#41132=CARTESIAN_POINT('Ctrl Pts',(-6.729655440052,3.66832849375325,8.81850134816314));
#41133=CARTESIAN_POINT('Ctrl Pts',(-7.66451426467329,0.0108335831259308,
8.93730872935627));
#41134=CARTESIAN_POINT('Ctrl Pts',(-6.73999869470739,-3.64928950279998,
9.05611611054938));
#41135=CARTESIAN_POINT('Ctrl Pts',(-4.18039177260559,-6.42411246067774,
9.17492349174251));
#41136=CARTESIAN_POINT('Ctrl Pts',(-0.606641859453193,-7.6404765515158,
9.29373087293563));
#41137=CARTESIAN_POINT('Ctrl Pts',(3.11427645879316,-7.00329768167184,9.41253825412875));
#41138=CARTESIAN_POINT('Ctrl Pts',(6.07968624705544,-4.66715238847722,9.53134563532187));
#41139=CARTESIAN_POINT('Ctrl Pts',(7.57019331551951,-1.19877831377079,9.650153016515));
#41140=CARTESIAN_POINT('Ctrl Pts',(7.2242077992116,2.5604136294189,9.76896039770811));
#41141=CARTESIAN_POINT('Ctrl Pts',(5.12566412472484,5.6984615081978,9.88776777890124));
#41142=CARTESIAN_POINT('Ctrl Pts',(1.78365892095447,7.4540899601228,10.0065751600944));
#41143=CARTESIAN_POINT('Ctrl Pts',(-1.9910533809796,7.40139194435702,10.1253825412875));
#41144=CARTESIAN_POINT('Ctrl Pts',(-5.28274568360125,5.55315174673762,10.2441899224806));
#41145=CARTESIAN_POINT('Ctrl Pts',(-7.29286922426337,2.35774357335561,10.3629973036737));
#41146=CARTESIAN_POINT('Ctrl Pts',(-7.53377767439077,-1.40964188102651,
10.4818046848669));
#41147=CARTESIAN_POINT('Ctrl Pts',(-5.94702779960401,-4.83505497700517,
10.60061206606));
#41148=CARTESIAN_POINT('Ctrl Pts',(-2.91755750801408,-7.08750692890673,
10.7194194472531));
#41149=CARTESIAN_POINT('Ctrl Pts',(0.819698239734408,-7.62056369802859,
10.8382268284462));
#41150=CARTESIAN_POINT('Ctrl Pts',(4.35809912656678,-6.30490826919325,10.9570342096394));
#41151=CARTESIAN_POINT('Ctrl Pts',(6.83924607068397,-3.45971233838136,11.0758415908324));
#41152=CARTESIAN_POINT('Ctrl Pts',(7.66122472541418,0.224793209818121,11.1946489720256));
#41153=CARTESIAN_POINT('Ctrl Pts',(6.62462701184582,3.85476500354751,11.3134563532187));
#41154=CARTESIAN_POINT('Ctrl Pts',(3.98092656328132,6.54958929855679,11.4322637344118));
#41155=CARTESIAN_POINT('Ctrl Pts',(0.37147242603168,7.65551464724345,11.5510711156049));
#41156=CARTESIAN_POINT('Ctrl Pts',(-3.32809913867807,6.90424886597847,11.6698784967981));
#41157=CARTESIAN_POINT('Ctrl Pts',(-6.22028981925211,4.47804542771158,11.7886858779912));
#41158=CARTESIAN_POINT('Ctrl Pts',(-7.60346802337159,0.965489651854728,
11.9074932591843));
#41159=CARTESIAN_POINT('Ctrl Pts',(-7.1420813670361,-2.78128928681395,12.0263006403774));
#41160=CARTESIAN_POINT('Ctrl Pts',(-4.94806001372185,-5.85334077701174,
12.1451080215706));
#41161=CARTESIAN_POINT('Ctrl Pts',(-1.55366307038099,-7.50539989050869,
12.2639154027637));
#41162=CARTESIAN_POINT('Ctrl Pts',(2.21764514742269,-7.33668495841004,12.3827227839568));
#41163=CARTESIAN_POINT('Ctrl Pts',(5.45096316026706,-5.38812551727601,12.5015301651499));
#41164=CARTESIAN_POINT('Ctrl Pts',(7.3619039130341,-2.13243253797661,12.6203375463431));
#41165=CARTESIAN_POINT('Ctrl Pts',(7.48688159171922,1.64057808329635,12.7391449275362));
#41166=CARTESIAN_POINT('Ctrl Pts',(5.79557868824736,5.01559284585168,12.8579523087293));
#41167=CARTESIAN_POINT('Ctrl Pts',(2.69829427965856,7.17384783520105,12.9767596899224));
#41168=CARTESIAN_POINT('Ctrl Pts',(-1.05357962331965,7.59176372731423,13.0955670711155));
#41169=CARTESIAN_POINT('Ctrl Pts',(-4.54986751928669,6.16795028626218,13.2143744523087));
#41170=CARTESIAN_POINT('Ctrl Pts',(-6.94236496891693,3.24782927505195,13.3331818335018));
#41171=CARTESIAN_POINT('Ctrl Pts',(-7.65070621468871,-0.460214393981673,
13.4519892146949));
#41172=CARTESIAN_POINT('Ctrl Pts',(-6.5029675097238,-4.05658315308385,13.570796595888));
#41173=CARTESIAN_POINT('Ctrl Pts',(-3.77774850024675,-6.66890133033136,
13.6896039770811));
#41174=CARTESIAN_POINT('Ctrl Pts',(-0.135853092147427,-7.66326421444017,
13.8084113582743));
#41175=CARTESIAN_POINT('Ctrl Pts',(3.53857938449235,-6.79877593351919,13.9272187394674));
#41176=CARTESIAN_POINT('Ctrl Pts',(6.3554303005832,-4.2844965243615,14.0460261206605));
#41177=CARTESIAN_POINT('Ctrl Pts',(7.20405402043916,-1.91602384960365,14.1252310414559));
#41178=CARTESIAN_POINT('Ctrl Pts',(7.32044999771583,-0.701660766284081,
14.1648335018536));
#41179=CARTESIAN_POINT('Ctrl Pts',(-3.33032948543731,6.87538113622997,-0.164833501853638));
#41180=CARTESIAN_POINT('Ctrl Pts',(-4.47086169837431,6.32292477307365,-0.12523104145593));
#41181=CARTESIAN_POINT('Ctrl Pts',(-6.47056832539346,4.6400650828852,-0.0460261206605157));
#41182=CARTESIAN_POINT('Ctrl Pts',(-7.900576802617,0.98770468599294,0.0727812605326066));
#41183=CARTESIAN_POINT('Ctrl Pts',(-7.41382533207128,-2.90327045442965,
0.191588641725729));
#41184=CARTESIAN_POINT('Ctrl Pts',(-5.12857766773546,-6.09041490475487,
0.310396022918851));
#41185=CARTESIAN_POINT('Ctrl Pts',(-1.59912968769544,-7.79980630787381,
0.429203404111974));
#41186=CARTESIAN_POINT('Ctrl Pts',(2.31824314590249,-7.61712832309403,0.548010785305095));
#41187=CARTESIAN_POINT('Ctrl Pts',(5.67322965321975,-5.58650714481864,0.666818166498218));
#41188=CARTESIAN_POINT('Ctrl Pts',(7.65191360348882,-2.20065900033317,0.78562554769134));
#41189=CARTESIAN_POINT('Ctrl Pts',(7.77428219202533,1.71907523767275,0.904432928884463));
#41190=CARTESIAN_POINT('Ctrl Pts',(6.01064610428973,5.22176150653328,1.02324031007758));
#41191=CARTESIAN_POINT('Ctrl Pts',(2.78885667027882,7.45767785271547,1.14204769127071));
#41192=CARTESIAN_POINT('Ctrl Pts',(-1.10949630295707,7.8843950949722,1.26085507246383));
#41193=CARTESIAN_POINT('Ctrl Pts',(-4.73869064778711,6.39839704652136,1.37966245365695));
#41194=CARTESIAN_POINT('Ctrl Pts',(-7.21830144782795,3.36017798602418,1.49846983485007));
#41195=CARTESIAN_POINT('Ctrl Pts',(-7.94678690378614,-0.493203838785206,
1.61727721604319));
#41196=CARTESIAN_POINT('Ctrl Pts',(-6.74741999655458,-4.22693692955293,
1.73608459723632));
#41197=CARTESIAN_POINT('Ctrl Pts',(-3.91116135495011,-6.93523532019726,
1.85489197842944));
#41198=CARTESIAN_POINT('Ctrl Pts',(-0.126073735251096,-7.96107892933453,
1.97369935962256));
#41199=CARTESIAN_POINT('Ctrl Pts',(3.6895987704621,-7.0556029587033,2.09250674081569));
#41200=CARTESIAN_POINT('Ctrl Pts',(6.61019231182172,-4.43847156569197,2.21131412200881));
#41201=CARTESIAN_POINT('Ctrl Pts',(7.92718490754252,-0.744588256569963,
2.33012150320193));
#41202=CARTESIAN_POINT('Ctrl Pts',(7.32108047037813,3.12992858919279,2.44892888439505));
#41203=CARTESIAN_POINT('Ctrl Pts',(4.93891702987685,6.24513977458459,2.56773626558817));
#41204=CARTESIAN_POINT('Ctrl Pts',(1.35859600940177,7.84531000736881,2.6865436467813));
#41205=CARTESIAN_POINT('Ctrl Pts',(-2.55131388583866,7.54224566600566,2.80535102797442));
#41206=CARTESIAN_POINT('Ctrl Pts',(-5.84228727083374,5.40946870539838,2.92415840916754));
#41207=CARTESIAN_POINT('Ctrl Pts',(-7.71594978886729,1.96438058571516,3.04296579036067));
#41208=CARTESIAN_POINT('Ctrl Pts',(-7.71775990088224,-1.95725684114341,
3.16177317155378));
#41209=CARTESIAN_POINT('Ctrl Pts',(-5.84727848237734,-5.40407314711093,
3.28058055274691));
#41210=CARTESIAN_POINT('Ctrl Pts',(-2.55827535294654,-7.53988723048059,
3.39938793394003));
#41211=CARTESIAN_POINT('Ctrl Pts',(1.3513531052808,-7.84656083992666,3.51819531513315));
#41212=CARTESIAN_POINT('Ctrl Pts',(4.93314978249241,-6.24969642889428,3.63700269632627));
#41213=CARTESIAN_POINT('Ctrl Pts',(7.31818798637123,-3.13668564347232,3.7558100775194));
#41214=CARTESIAN_POINT('Ctrl Pts',(7.92786888948117,0.737270032641113,3.87461745871252));
#41215=CARTESIAN_POINT('Ctrl Pts',(6.61428682931535,4.43236753545784,3.99342483990565));
#41216=CARTESIAN_POINT('Ctrl Pts',(3.69611051252854,7.05219393586209,4.11223222109876));
#41217=CARTESIAN_POINT('Ctrl Pts',(-0.118724484670133,7.9611919162004,4.23103960229189));
#41218=CARTESIAN_POINT('Ctrl Pts',(-3.90475749139907,6.93884292682844,4.349846983485));
#41219=CARTESIAN_POINT('Ctrl Pts',(-6.74351506150395,4.2331639284469,4.46865436467813));
#41220=CARTESIAN_POINT('Ctrl Pts',(-7.94632822575575,0.500539667151168,
4.58746174587125));
#41221=CARTESIAN_POINT('Ctrl Pts',(-7.22140028029939,-3.35351311634923,
4.70626912706438));
#41222=CARTESIAN_POINT('Ctrl Pts',(-4.7445952672849,-6.39401970434032,4.82507650825749));
#41223=CARTESIAN_POINT('Ctrl Pts',(-1.11677420184678,-7.88336778362672,
4.94388388945062));
#41224=CARTESIAN_POINT('Ctrl Pts',(2.78197092788859,-7.46024865444962,5.06269127064373));
#41225=CARTESIAN_POINT('Ctrl Pts',(6.00582325539593,-5.22730898788083,5.18149865183687));
#41226=CARTESIAN_POINT('Ctrl Pts',(7.77269167056723,-1.72624923580848,5.30030603302998));
#41227=CARTESIAN_POINT('Ctrl Pts',(7.65394237139929,2.19359030020036,5.41911341422311));
#41228=CARTESIAN_POINT('Ctrl Pts',(5.67838336823999,5.58127535184656,5.53792079541623));
#41229=CARTESIAN_POINT('Ctrl Pts',(2.32527579866739,7.6149697760376,5.65672817660936));
#41230=CARTESIAN_POINT('Ctrl Pts',(-1.5919325255118,7.80130906092382,5.77553555780247));
#41231=CARTESIAN_POINT('Ctrl Pts',(-5.12294565536668,6.0950881898455,5.8943429389956));
#41232=CARTESIAN_POINT('Ctrl Pts',(-7.41115674356387,2.91022816152997,6.01315032018872));
#41233=CARTESIAN_POINT('Ctrl Pts',(-7.90145675646063,-0.980639258655962,
6.13195770138184));
#41234=CARTESIAN_POINT('Ctrl Pts',(-6.47490126285554,-4.63360829873503,
6.25076508257496));
#41235=CARTESIAN_POINT('Ctrl Pts',(-3.47756578243197,-7.1624861925656,6.36957246376809));
#41236=CARTESIAN_POINT('Ctrl Pts',(0.363410475222534,-7.95377929391638,
6.48837984496121));
#41237=CARTESIAN_POINT('Ctrl Pts',(4.11622509483713,-6.81552369216537,6.60718722615433));
#41238=CARTESIAN_POINT('Ctrl Pts',(6.87046325162571,-4.02385473618211,6.72599460734745));
#41239=CARTESIAN_POINT('Ctrl Pts',(7.95795998059733,-0.256017923289772,
6.84480198854058));
#41240=CARTESIAN_POINT('Ctrl Pts',(7.11489379193279,3.57392760969647,6.96360936973369));
#41241=CARTESIAN_POINT('Ctrl Pts',(4.54578849888529,6.53685544839694,7.08241675092683));
#41242=CARTESIAN_POINT('Ctrl Pts',(0.873896721768728,7.91397351205552,7.20122413211994));
#41243=CARTESIAN_POINT('Ctrl Pts',(-3.00999820804074,7.37119956434678,7.32003151331307));
#41244=CARTESIAN_POINT('Ctrl Pts',(-6.16368201128471,5.04020796134442,7.43883889450619));
#41245=CARTESIAN_POINT('Ctrl Pts',(-7.82208612524901,1.48648608436854,7.5576462756993));
#41246=CARTESIAN_POINT('Ctrl Pts',(-7.5828896671093,-2.42785018612792,7.67645365689243));
#41247=CARTESIAN_POINT('Ctrl Pts',(-5.50412055020522,-5.75320164766046,
7.79526103808555));
#41248=CARTESIAN_POINT('Ctrl Pts',(-2.09007819061915,-7.68285398708923,
7.91406841927868));
#41249=CARTESIAN_POINT('Ctrl Pts',(1.83100711208394,-7.74868280324678,8.0328758004718));
#41250=CARTESIAN_POINT('Ctrl Pts',(5.30789887258074,-5.93471834110859,8.15168318166492));
#41251=CARTESIAN_POINT('Ctrl Pts',(7.49711982812857,-2.6810196777562,8.27049056285805));
#41252=CARTESIAN_POINT('Ctrl Pts',(7.86757547641812,1.22308149879663,8.38929794405116));
#41253=CARTESIAN_POINT('Ctrl Pts',(6.32939505421858,4.83046897075924,8.5081053252443));
#41254=CARTESIAN_POINT('Ctrl Pts',(3.25573375343499,7.26600784176417,8.6269127064374));
#41255=CARTESIAN_POINT('Ctrl Pts',(-0.607752938454231,7.93884806477834,
8.74572008763054));
#41256=CARTESIAN_POINT('Ctrl Pts',(-4.32380168281358,6.68576182925573,8.86452746882365));
#41257=CARTESIAN_POINT('Ctrl Pts',(-6.99091687983101,3.81074184498614,8.98333485001678));
#41258=CARTESIAN_POINT('Ctrl Pts',(-7.96206917663469,0.0112541689272012,
9.10214223120989));
#41259=CARTESIAN_POINT('Ctrl Pts',(-7.00166168455497,-3.79096371452819,
9.22094961240303));
#41260=CARTESIAN_POINT('Ctrl Pts',(-4.34268465417737,-6.67351198576931,
9.33975699359614));
#41261=CARTESIAN_POINT('Ctrl Pts',(-0.63019315818504,-7.93709826153181,
9.45856437478927));
#41262=CARTESIAN_POINT('Ctrl Pts',(3.23518017500003,-7.2751825726315,9.57737175598238));
#41263=CARTESIAN_POINT('Ctrl Pts',(6.31571431661408,-4.8483424900424,9.69617913717552));
#41264=CARTESIAN_POINT('Ctrl Pts',(7.86408646096156,-1.24531777645527,9.81498651836863));
#41265=CARTESIAN_POINT('Ctrl Pts',(7.50466895323321,2.65981505601654,9.93379389956176));
#41266=CARTESIAN_POINT('Ctrl Pts',(5.32465475670866,5.91968951480514,10.0526012807549));
#41267=CARTESIAN_POINT('Ctrl Pts',(1.85290485812236,7.74347569354884,10.171408661948));
#41268=CARTESIAN_POINT('Ctrl Pts',(-2.06835087081773,7.6887318138313,10.2902160431411));
#41269=CARTESIAN_POINT('Ctrl Pts',(-5.48783460020011,5.76873847827063,10.4090234243343));
#41270=CARTESIAN_POINT('Ctrl Pts',(-7.57599598025021,2.44927686002859,10.5278308055273));
#41271=CARTESIAN_POINT('Ctrl Pts',(-7.82625707689805,-1.46436757548299,
10.6466381867205));
#41272=CARTESIAN_POINT('Ctrl Pts',(-6.17790574858239,-5.02276346163052,
10.7654455679136));
#41273=CARTESIAN_POINT('Ctrl Pts',(-3.03082412054307,-7.36266102575237,
10.8842529491067));
#41274=CARTESIAN_POINT('Ctrl Pts',(0.851520900523648,-7.91641234309075,
11.0030603302998));
#41275=CARTESIAN_POINT('Ctrl Pts',(4.52729103581818,-6.54968000034022,11.121867711493));
#41276=CARTESIAN_POINT('Ctrl Pts',(7.10476208281073,-3.59402670778684,11.2406750926861));
#41277=CARTESIAN_POINT('Ctrl Pts',(7.95865192953517,0.233520223878897,11.3594824738792));
#41278=CARTESIAN_POINT('Ctrl Pts',(6.88181099496819,4.00441626932297,11.4782898550723));
#41279=CARTESIAN_POINT('Ctrl Pts',(4.13547572480117,6.80386013684043,11.5970972362655));
#41280=CARTESIAN_POINT('Ctrl Pts',(0.385893880700171,7.952720172371,11.7159046174586));
#41281=CARTESIAN_POINT('Ctrl Pts',(-3.45730396653943,7.17228844324756,11.8347119986517));
#41282=CARTESIAN_POINT('Ctrl Pts',(-6.46177645827802,4.6518939413928,11.9535193798448));
#41283=CARTESIAN_POINT('Ctrl Pts',(-7.89865297315028,1.00297228655756,12.072326761038));
#41284=CARTESIAN_POINT('Ctrl Pts',(-7.41935417507103,-2.88926563864769,
12.1911341422311));
#41285=CARTESIAN_POINT('Ctrl Pts',(-5.14015562616646,-6.08058157002734,
12.3099415234242));
#41286=CARTESIAN_POINT('Ctrl Pts',(-1.61398001443781,-7.79677759906733,
12.4287489046173));
#41287=CARTESIAN_POINT('Ctrl Pts',(2.30373947562354,-7.62151274677366,12.5475562858105));
#41288=CARTESIAN_POINT('Ctrl Pts',(5.6625826846424,-5.59730553293856,12.6663636670036));
#41289=CARTESIAN_POINT('Ctrl Pts',(7.64771076198313,-2.21521870735279,12.7851710481967));
#41290=CARTESIAN_POINT('Ctrl Pts',(7.77754037529766,1.70426927758259,12.9039784293898));
#41291=CARTESIAN_POINT('Ctrl Pts',(6.02057701779519,5.21031024556484,13.022785810583));
#41292=CARTESIAN_POINT('Ctrl Pts',(2.80304856533202,7.45235389407376,13.141593191776));
#41293=CARTESIAN_POINT('Ctrl Pts',(-1.09448212297394,7.88649428811764,13.2604005729692));
#41294=CARTESIAN_POINT('Ctrl Pts',(-4.72650433962341,6.40740497850149,13.3792079541623));
#41295=CARTESIAN_POINT('Ctrl Pts',(-7.21188430514562,3.37391783339129,13.4980153353554));
#41296=CARTESIAN_POINT('Ctrl Pts',(-7.94772506487821,-0.47808102567622,
13.6168227165485));
#41297=CARTESIAN_POINT('Ctrl Pts',(-6.75542837782637,-4.21406948571987,
13.7356300977417));
#41298=CARTESIAN_POINT('Ctrl Pts',(-3.9244097997872,-6.92780414917955,13.8544374789348));
#41299=CARTESIAN_POINT('Ctrl Pts',(-0.141127236532553,-7.96077059643944,
13.9732448601279));
#41300=CARTESIAN_POINT('Ctrl Pts',(3.67595556266374,-7.06272079740548,14.092052241321));
#41301=CARTESIAN_POINT('Ctrl Pts',(6.60216341872522,-4.45083100324446,14.2108596225142));
#41302=CARTESIAN_POINT('Ctrl Pts',(7.48373275620681,-1.99040851224466,14.2900645433096));
#41303=CARTESIAN_POINT('Ctrl Pts',(7.60464750578597,-0.728900927934096,
14.3296670037073));
#41304=CARTESIAN_POINT('Ctrl Pts',(-3.45478907940187,7.13232482552818,0.));
#41305=CARTESIAN_POINT('Ctrl Pts',(-4.6379447554966,6.55922230860773,0.0396024603977074));
#41306=CARTESIAN_POINT('Ctrl Pts',(-6.71238353017122,4.81347153372149,0.118807381193122));
#41307=CARTESIAN_POINT('Ctrl Pts',(-8.19583364889584,1.02461674671041,0.237614762386245));
#41308=CARTESIAN_POINT('Ctrl Pts',(-7.69089151864192,-3.01177018801687,
0.356422143579367));
#41309=CARTESIAN_POINT('Ctrl Pts',(-5.32024059386133,-6.31802318478726,
0.475229524772489));
#41310=CARTESIAN_POINT('Ctrl Pts',(-1.65889165193879,-8.0912972039924,0.594036905965612));
#41311=CARTESIAN_POINT('Ctrl Pts',(2.40487949882547,-7.90179225872376,0.712844287158733));
#41312=CARTESIAN_POINT('Ctrl Pts',(5.88524707137462,-5.79528360791777,0.831651668351856));
#41313=CARTESIAN_POINT('Ctrl Pts',(7.93787751916342,-2.28290105080705,0.950459049544978));
#41314=CARTESIAN_POINT('Ctrl Pts',(8.06481921222603,1.78331975372163,1.0692664307381));
#41315=CARTESIAN_POINT('Ctrl Pts',(6.23527330015003,5.41690685768391,1.18807381193122));
#41316=CARTESIAN_POINT('Ctrl Pts',(2.89308058275538,7.73638287620525,1.30688119312434));
#41317=CARTESIAN_POINT('Ctrl Pts',(-1.15095990587534,8.17904720566199,1.42568857431747));
#41318=CARTESIAN_POINT('Ctrl Pts',(-4.91578288941853,6.63751509832866,1.54449595551059));
#41319=CARTESIAN_POINT('Ctrl Pts',(-7.488060602662,3.48575306489192,1.66330333670371));
#41320=CARTESIAN_POINT('Ctrl Pts',(-8.24377069343612,-0.511635633532653,
1.78211071789683));
#41321=CARTESIAN_POINT('Ctrl Pts',(-6.99958157899013,-4.38490413858326,
1.90091809908996));
#41322=CARTESIAN_POINT('Ctrl Pts',(-4.057327539496,-7.1944158534673,2.01972548028308));
#41323=CARTESIAN_POINT('Ctrl Pts',(-0.130785306874149,-8.25859683421376,
2.1385328614762));
#41324=CARTESIAN_POINT('Ctrl Pts',(3.82748481653407,-7.31928181788386,2.25734024266932));
#41325=CARTESIAN_POINT('Ctrl Pts',(6.85722548218955,-4.60434415316564,2.37614762386244));
#41326=CARTESIAN_POINT('Ctrl Pts',(8.22343614009745,-0.772414678096356,
2.49495500505557));
#41327=CARTESIAN_POINT('Ctrl Pts',(7.59468063718132,3.24689888989499,2.61376238624869));
#41328=CARTESIAN_POINT('Ctrl Pts',(5.12349204290518,6.47853036371263,2.73256976744181));
#41329=CARTESIAN_POINT('Ctrl Pts',(1.40936885588182,8.13850144752901,2.85137714863493));
#41330=CARTESIAN_POINT('Ctrl Pts',(-2.64666045490822,7.8241111202428,2.97018452982806));
#41331=CARTESIAN_POINT('Ctrl Pts',(-6.06062263516686,5.61162896659236,3.08899191102118));
#41332=CARTESIAN_POINT('Ctrl Pts',(-8.00430683641251,2.03779254424933,3.2077992922143));
#41333=CARTESIAN_POINT('Ctrl Pts',(-8.00618459512947,-2.03040257426028,
3.32660667340743));
#41334=CARTESIAN_POINT('Ctrl Pts',(-6.06580037605087,-5.60603176789764,
3.44541405460054));
#41335=CARTESIAN_POINT('Ctrl Pts',(-2.65388208287209,-7.82166454631306,
3.56422143579367));
#41336=CARTESIAN_POINT('Ctrl Pts',(1.40185527316581,-8.13979902564551,3.68302881698679));
#41337=CARTESIAN_POINT('Ctrl Pts',(5.11750926451368,-6.48325730728283,3.80183619817991));
#41338=CARTESIAN_POINT('Ctrl Pts',(7.59168005654716,-3.25390846580513,3.92064357937303));
#41339=CARTESIAN_POINT('Ctrl Pts',(8.22414568350524,0.764822960754067,4.03945096056616));
#41340=CARTESIAN_POINT('Ctrl Pts',(6.86147301817189,4.59801200582542,4.15825834175928));
#41341=CARTESIAN_POINT('Ctrl Pts',(3.83423991253207,7.31574539455554,4.27706572295241));
#41342=CARTESIAN_POINT('Ctrl Pts',(-0.123161403365499,8.25871404357459,
4.39587310414552));
#41343=CARTESIAN_POINT('Ctrl Pts',(-4.05068435360135,7.19815828197074,4.51468048533865));
#41344=CARTESIAN_POINT('Ctrl Pts',(-6.99553071044162,4.39136385011345,4.63348786653177));
#41345=CARTESIAN_POINT('Ctrl Pts',(-8.24329487389415,0.519245613217243,
4.75229524772489));
#41346=CARTESIAN_POINT('Ctrl Pts',(-7.49127524332387,-3.47883911866845,
4.87110262891801));
#41347=CARTESIAN_POINT('Ctrl Pts',(-4.92190817373296,-6.63297416806032,
4.98991001011114));
#41348=CARTESIAN_POINT('Ctrl Pts',(-1.15850979116904,-8.17798150209332,
5.10871739130425));
#41349=CARTESIAN_POINT('Ctrl Pts',(2.88593750945964,-7.73904975279968,5.22752477249739));
#41350=CARTESIAN_POINT('Ctrl Pts',(6.23027021389002,-5.42266165703982,5.34633215369049));
#41351=CARTESIAN_POINT('Ctrl Pts',(8.06316925050661,-1.79076185532853,5.46513953488364));
#41352=CARTESIAN_POINT('Ctrl Pts',(7.93998210528692,2.27556818235326,5.58394691607674));
#41353=CARTESIAN_POINT('Ctrl Pts',(5.89059338874298,5.78985629470304,5.70275429726988));
#41354=CARTESIAN_POINT('Ctrl Pts',(2.41217497276513,7.89955304340571,5.82156167846299));
#41355=CARTESIAN_POINT('Ctrl Pts',(-1.65142552060749,8.09285611726176,5.94036905965612));
#41356=CARTESIAN_POINT('Ctrl Pts',(-5.31439810442841,6.32287111781213,6.05917644084924));
#41357=CARTESIAN_POINT('Ctrl Pts',(-7.68812320083037,3.01898791545586,6.17798382204235));
#41358=CARTESIAN_POINT('Ctrl Pts',(-8.19674648798357,-1.01728727336192,
6.29679120323548));
#41359=CARTESIAN_POINT('Ctrl Pts',(-6.71687839624717,-4.8067734495026,6.4155985844286));
#41360=CARTESIAN_POINT('Ctrl Pts',(-3.60752782587519,-7.43015944447703,
6.53440596562173));
#41361=CARTESIAN_POINT('Ctrl Pts',(0.376991690050199,-8.25102440006379,
6.65321334681485));
#41362=CARTESIAN_POINT('Ctrl Pts',(4.2700548303664,-7.07023041565686,6.77202072800797));
#41363=CARTESIAN_POINT('Ctrl Pts',(7.12722315192535,-4.17423244770513,6.89082810920109));
#41364=CARTESIAN_POINT('Ctrl Pts',(8.25536132551003,-0.265585711377908,
7.00963549039422));
#41365=CARTESIAN_POINT('Ctrl Pts',(7.38078844179166,3.70749084453752,7.12844287158733));
#41366=CARTESIAN_POINT('Ctrl Pts',(4.71567168710858,6.78114790608622,7.24725025278046));
#41367=CARTESIAN_POINT('Ctrl Pts',(0.90655560180866,8.20973101420773,7.36605763397358));
#41368=CARTESIAN_POINT('Ctrl Pts',(-3.12248652381999,7.64667275966336,7.4848650151667));
#41369=CARTESIAN_POINT('Ctrl Pts',(-6.39402839707196,5.22856837406304,7.60367239635983));
#41370=CARTESIAN_POINT('Ctrl Pts',(-8.1144096528043,1.54203838191253,7.72247977755296));
#41371=CARTESIAN_POINT('Ctrl Pts',(-7.86627405089878,-2.51858272466308,
7.84128715874606));
#41372=CARTESIAN_POINT('Ctrl Pts',(-5.70981809809234,-5.96820774366244,
7.9600945399392));
#41373=CARTESIAN_POINT('Ctrl Pts',(-2.16818766420013,-7.96997419303383,
8.07890192113231));
#41374=CARTESIAN_POINT('Ctrl Pts',(1.89943469641536,-8.03826313446309,8.19770930232545));
#41375=CARTESIAN_POINT('Ctrl Pts',(5.50626331110705,-6.1565079983357,8.31651668351855));
#41376=CARTESIAN_POINT('Ctrl Pts',(7.7772988596006,-2.78121355405694,8.43532406471168));
#41377=CARTESIAN_POINT('Ctrl Pts',(8.16159901179575,1.26878995719133,8.55413144590481));
#41378=CARTESIAN_POINT('Ctrl Pts',(6.56593439422505,5.01099111110242,8.67293882709792));
#41379=CARTESIAN_POINT('Ctrl Pts',(3.37740558884383,7.53754985875791,8.79174620829106));
#41380=CARTESIAN_POINT('Ctrl Pts',(-0.630465611263786,8.2355351676639,8.91055358948416));
#41381=CARTESIAN_POINT('Ctrl Pts',(-4.48538887836867,6.93561915005586,9.0293609706773));
#41382=CARTESIAN_POINT('Ctrl Pts',(-7.25217831961001,3.95315519621903,9.14816835187041));
#41383=CARTESIAN_POINT('Ctrl Pts',(-8.25962408859611,0.0116747547284766,
9.26697573306354));
#41384=CARTESIAN_POINT('Ctrl Pts',(-7.26332467440254,-3.93263792625641,
9.38578311425666));
#41385=CARTESIAN_POINT('Ctrl Pts',(-4.50497753574917,-6.92291151086089,
9.50459049544978));
#41386=CARTESIAN_POINT('Ctrl Pts',(-0.653744456916887,-8.23371997154782,
9.62339787664291));
#41387=CARTESIAN_POINT('Ctrl Pts',(3.35608389120691,-7.54706746359117,9.74220525783602));
#41388=CARTESIAN_POINT('Ctrl Pts',(6.55174238617272,-5.02953259160757,9.86101263902915));
#41389=CARTESIAN_POINT('Ctrl Pts',(8.15797960640361,-1.29185723913975,9.97982002022227));
#41390=CARTESIAN_POINT('Ctrl Pts',(7.78513010725481,2.75921648261417,10.0986274014154));
#41391=CARTESIAN_POINT('Ctrl Pts',(5.52364538869249,6.14091752141248,10.2174347826085));
#41392=CARTESIAN_POINT('Ctrl Pts',(1.92215079529024,8.03286142697488,10.3362421638016));
#41393=CARTESIAN_POINT('Ctrl Pts',(-2.14564836065585,7.9760716833056,10.4550495449947));
#41394=CARTESIAN_POINT('Ctrl Pts',(-5.69292351679898,5.98432520980362,10.5738569261879));
#41395=CARTESIAN_POINT('Ctrl Pts',(-7.85912273623703,2.54081014670158,10.692664307381));
#41396=CARTESIAN_POINT('Ctrl Pts',(-8.11873647940535,-1.51909326993947,
10.8114716885741));
#41397=CARTESIAN_POINT('Ctrl Pts',(-6.40878369756076,-5.21047194625588,
10.9302790697672));
#41398=CARTESIAN_POINT('Ctrl Pts',(-3.14409073307205,-7.637815122598,11.0490864509604));
#41399=CARTESIAN_POINT('Ctrl Pts',(0.883343561312894,-8.21226098815292,
11.1678938321535));
#41400=CARTESIAN_POINT('Ctrl Pts',(4.69648294506956,-6.79445173148717,11.2867012133466));
#41401=CARTESIAN_POINT('Ctrl Pts',(7.37027809493751,-3.72834107719234,11.4055085945397));
#41402=CARTESIAN_POINT('Ctrl Pts',(8.25607913365615,0.242247237939676,11.5243159757329));
#41403=CARTESIAN_POINT('Ctrl Pts',(7.13899497809059,4.15406753509843,11.643123356926));
#41404=CARTESIAN_POINT('Ctrl Pts',(4.290024886321,7.05813097512407,11.7619307381191));
#41405=CARTESIAN_POINT('Ctrl Pts',(0.400315335368676,8.24992569749855,11.8807381193122));
#41406=CARTESIAN_POINT('Ctrl Pts',(-3.5865087944008,7.44032802051665,11.9995455005053));
#41407=CARTESIAN_POINT('Ctrl Pts',(-6.7032630973039,4.82574245507403,12.1183528816985));
#41408=CARTESIAN_POINT('Ctrl Pts',(-8.19383792292899,1.04045492126039,12.2371602628916));
#41409=CARTESIAN_POINT('Ctrl Pts',(-7.69662698310595,-2.99724199048142,
12.3559676440847));
#41410=CARTESIAN_POINT('Ctrl Pts',(-5.33225123861107,-6.30782236304295,
12.4747750252778));
#41411=CARTESIAN_POINT('Ctrl Pts',(-1.67429695849463,-8.08815530762596,
12.593582406471));
#41412=CARTESIAN_POINT('Ctrl Pts',(2.38983380382439,-7.90634053513729,12.7123897876641));
#41413=CARTESIAN_POINT('Ctrl Pts',(5.87420220901772,-5.80648554860111,12.8311971688572));
#41414=CARTESIAN_POINT('Ctrl Pts',(7.93351761093217,-2.29800487672896,12.9500045500503));
#41415=CARTESIAN_POINT('Ctrl Pts',(8.06819915887609,1.76796047186882,13.0688119312434));
#41416=CARTESIAN_POINT('Ctrl Pts',(6.24557534734301,5.40502764527801,13.1876193124366));
#41417=CARTESIAN_POINT('Ctrl Pts',(2.90780285100547,7.73085995294645,13.3064266936297));
#41418=CARTESIAN_POINT('Ctrl Pts',(-1.13538462262823,8.18122484892105,13.4252340748228));
#41419=CARTESIAN_POINT('Ctrl Pts',(-4.90314115996014,6.6468596707408,13.5440414560159));
#41420=CARTESIAN_POINT('Ctrl Pts',(-7.48140364137431,3.50000639173062,13.6628488372091));
#41421=CARTESIAN_POINT('Ctrl Pts',(-8.24474391506772,-0.495947657370763,
13.7816562184022));
#41422=CARTESIAN_POINT('Ctrl Pts',(-7.00788924592892,-4.3715558183559,13.9004635995953));
#41423=CARTESIAN_POINT('Ctrl Pts',(-4.07107109932766,-7.18670696802772,
14.0192709807884));
#41424=CARTESIAN_POINT('Ctrl Pts',(-0.146401380917679,-8.25827697843872,
14.1380783619815));
#41425=CARTESIAN_POINT('Ctrl Pts',(3.81333174083514,-7.32666566129177,14.2568857431747));
#41426=CARTESIAN_POINT('Ctrl Pts',(6.84889653686724,-4.61716548212742,14.3756931243678));
#41427=CARTESIAN_POINT('Ctrl Pts',(7.76341149197447,-2.06479317488566,14.4548980451632));
#41428=CARTESIAN_POINT('Ctrl Pts',(7.88884501385612,-0.756141089584111,
14.4945005055609));
#41429=CARTESIAN_POINT('',(-4.44937994724887,-6.55809752024317,14.));
#41430=CARTESIAN_POINT('Ctrl Pts',(-4.44940638321902,-6.5584391708898,14.));
#41431=CARTESIAN_POINT('Ctrl Pts',(-4.26689467651366,-6.66907515586647,
14.));
#41432=CARTESIAN_POINT('Ctrl Pts',(-4.08028782328584,-6.77205836122323,
14.));
#41433=CARTESIAN_POINT('Ctrl Pts',(-3.88997616949827,-6.86706524648209,
14.));
#41434=CARTESIAN_POINT('Ctrl Pts',(-3.70514829807453,-6.95933453227472,
14.));
#41435=CARTESIAN_POINT('Ctrl Pts',(-3.51682535429916,-7.04408071741637,
14.));
#41436=CARTESIAN_POINT('Ctrl Pts',(-3.32549660258128,-7.12123542969775,
14.));
#41437=CARTESIAN_POINT('Ctrl Pts',(-3.13345808093299,-7.19867636187171,
14.));
#41438=CARTESIAN_POINT('Ctrl Pts',(-2.93839070791496,-7.26846953339858,
14.));
#41439=CARTESIAN_POINT('Ctrl Pts',(-2.7407745157787,-7.33049546272157,14.));
#41440=CARTESIAN_POINT('Ctrl Pts',(-2.54412235497741,-7.39221881087042,
14.));
#41441=CARTESIAN_POINT('Ctrl Pts',(-2.34494548635082,-7.44625059009398,
14.));
#41442=CARTESIAN_POINT('Ctrl Pts',(-2.1437128994453,-7.49242178207046,14.));
#41443=CARTESIAN_POINT('Ctrl Pts',(-1.97939455606432,-7.53012329897767,
14.));
#41444=CARTESIAN_POINT('Ctrl Pts',(-1.81370528628452,-7.56258270331728,
14.));
#41445=CARTESIAN_POINT('Ctrl Pts',(-1.64690325240232,-7.58968182048372,
14.));
#41446=CARTESIAN_POINT('Ctrl Pts',(-1.61532958921609,-7.59481136463941,
14.));
#41447=CARTESIAN_POINT('Ctrl Pts',(-1.58371164972916,-7.59974937840371,
14.));
#41448=CARTESIAN_POINT('Ctrl Pts',(-1.55207992279835,-7.60449085285328,
14.));
#41449=CARTESIAN_POINT('Ctrl Pts',(-1.34986154646332,-7.63480261125719,
14.));
#41450=CARTESIAN_POINT('Ctrl Pts',(-1.14687126288046,-7.65712242315947,
14.));
#41451=CARTESIAN_POINT('Ctrl Pts',(-0.943573958042012,-7.67137342384431,
14.));
#41452=CARTESIAN_POINT('Ctrl Pts',(-0.741135905208625,-7.68556419155694,
14.));
#41453=CARTESIAN_POINT('Ctrl Pts',(-0.538392736482371,-7.69175426249507,
14.));
#41454=CARTESIAN_POINT('Ctrl Pts',(-0.335799622499727,-7.68981648545354,
14.));
#41455=CARTESIAN_POINT('Ctrl Pts',(-0.269283413955203,-7.689180266486,14.));
#41456=CARTESIAN_POINT('Ctrl Pts',(-0.202783393657834,-7.68766747636142,
14.));
#41457=CARTESIAN_POINT('Ctrl Pts',(-0.136315770622695,-7.68527238702149,
14.));
#41458=CARTESIAN_POINT('Ctrl Pts',(0.0672666969070029,-7.67793651166577,
14.));
#41459=CARTESIAN_POINT('Ctrl Pts',(0.270546320464125,-7.66232728574139,
14.));
#41460=CARTESIAN_POINT('Ctrl Pts',(0.473045266450486,-7.63856454842076,
14.));
#41461=CARTESIAN_POINT('Ctrl Pts',(0.674485516628634,-7.61492604636601,
14.));
#41462=CARTESIAN_POINT('Ctrl Pts',(0.875153886334405,-7.58321879930691,
14.));
#41463=CARTESIAN_POINT('Ctrl Pts',(1.07456032484331,-7.5435134068963,14.));
#41464=CARTESIAN_POINT('Ctrl Pts',(1.13439659455426,-7.53159893418906,14.));
#41465=CARTESIAN_POINT('Ctrl Pts',(1.19411906441983,-7.51896397318094,14.));
#41466=CARTESIAN_POINT('Ctrl Pts',(1.2537140095434,-7.50560964743804,14.));
#41467=CARTESIAN_POINT('Ctrl Pts',(1.28943769992771,-7.49760450879513,14.));
#41468=CARTESIAN_POINT('Ctrl Pts',(1.32511556208652,-7.48934087383794,14.));
#41469=CARTESIAN_POINT('Ctrl Pts',(1.3607445945539,-7.48081892436368,14.));
#41470=CARTESIAN_POINT('Ctrl Pts',(1.38465203572509,-7.47510061006742,14.));
#41471=CARTESIAN_POINT('Ctrl Pts',(1.40852886519995,-7.46926803693634,14.));
#41472=CARTESIAN_POINT('Ctrl Pts',(1.43237022598248,-7.46332253618824,14.));
#41473=CARTESIAN_POINT('Ctrl Pts',(1.62769405447016,-7.41461315340646,14.));
#41474=CARTESIAN_POINT('Ctrl Pts',(1.82072584398294,-7.35830742188736,14.));
#41475=CARTESIAN_POINT('Ctrl Pts',(2.01102139547125,-7.29457501043332,14.));
#41476=CARTESIAN_POINT('Ctrl Pts',(2.20118757483255,-7.23088592735752,14.));
#41477=CARTESIAN_POINT('Ctrl Pts',(2.38862189549973,-7.15977999794911,14.));
#41478=CARTESIAN_POINT('Ctrl Pts',(2.5728645161657,-7.08137730080356,14.));
#41479=CARTESIAN_POINT('Ctrl Pts',(2.75481210731953,-7.00395123166693,14.));
#41480=CARTESIAN_POINT('Ctrl Pts',(2.93364759189136,-6.91940872604078,14.));
#41481=CARTESIAN_POINT('Ctrl Pts',(3.10890286121801,-6.8278218581436,14.));
#41482=CARTESIAN_POINT('Ctrl Pts',(3.22552198713502,-6.76687772493333,14.));
#41483=CARTESIAN_POINT('Ctrl Pts',(3.34055530131138,-6.70281353757012,14.));
#41484=CARTESIAN_POINT('Ctrl Pts',(3.4538566828235,-6.63564064344417,14.));
#41485=CARTESIAN_POINT('Ctrl Pts',(3.58559135870223,-6.55753921769436,14.));
#41486=CARTESIAN_POINT('Ctrl Pts',(3.7149850616138,-6.4752353085306,14.));
#41487=CARTESIAN_POINT('Ctrl Pts',(3.84185984001097,-6.38886310040951,14.));
#41488=CARTESIAN_POINT('Ctrl Pts',(3.8806004845034,-6.36248973407842,14.));
#41489=CARTESIAN_POINT('Ctrl Pts',(3.9191061724772,-6.33573698326292,14.));
#41490=CARTESIAN_POINT('Ctrl Pts',(3.95737155880359,-6.30860848485213,14.));
#41491=CARTESIAN_POINT('Ctrl Pts',(3.97728091824068,-6.29449361296134,14.));
#41492=CARTESIAN_POINT('Ctrl Pts',(3.99712719655925,-6.28027559103114,14.));
#41493=CARTESIAN_POINT('Ctrl Pts',(4.01690323841346,-6.26595955416571,14.));
#41494=CARTESIAN_POINT('Ctrl Pts',(4.17634630198718,-6.1505374291072,14.));
#41495=CARTESIAN_POINT('Ctrl Pts',(4.33089390508824,-6.028990302188,14.));
#41496=CARTESIAN_POINT('Ctrl Pts',(4.48025060970871,-5.90169460830379,14.));
#41497=CARTESIAN_POINT('Ctrl Pts',(4.63343708131297,-5.77113483031398,14.));
#41498=CARTESIAN_POINT('Ctrl Pts',(4.78116368530107,-5.63452748859809,14.));
#41499=CARTESIAN_POINT('Ctrl Pts',(4.92307572794479,-5.49223569146564,14.));
#41500=CARTESIAN_POINT('Ctrl Pts',(5.06165950670547,-5.35328106460028,14.));
#41501=CARTESIAN_POINT('Ctrl Pts',(5.19469858019819,-5.2089048176019,14.));
#41502=CARTESIAN_POINT('Ctrl Pts',(5.32182205546165,-5.05941318879982,14.));
#41503=CARTESIAN_POINT('Ctrl Pts',(5.45352507612924,-4.9045362155504,14.));
#41504=CARTESIAN_POINT('Ctrl Pts',(5.57887944752641,-4.74416823716401,14.));
#41505=CARTESIAN_POINT('Ctrl Pts',(5.69741932593274,-4.57862308077917,14.));
#41506=CARTESIAN_POINT('Ctrl Pts',(5.75668926513591,-4.49585050258675,14.));
#41507=CARTESIAN_POINT('Ctrl Pts',(5.81425468118815,-4.41178326119413,14.));
#41508=CARTESIAN_POINT('Ctrl Pts',(5.87005158672204,-4.32645875741048,14.));
#41509=CARTESIAN_POINT('Ctrl Pts',(5.89510682009737,-4.2881443502856,14.));
#41510=CARTESIAN_POINT('Ctrl Pts',(5.91980539685357,-4.24957641531242,14.));
#41511=CARTESIAN_POINT('Ctrl Pts',(5.94414125164539,-4.21075828020098,14.));
#41512=CARTESIAN_POINT('Ctrl Pts',(5.95731830661959,-4.18973955270054,14.));
#41513=CARTESIAN_POINT('Ctrl Pts',(5.97038804733471,-4.168648934416,14.));
#41514=CARTESIAN_POINT('Ctrl Pts',(5.98334356622436,-4.14749695834229,14.));
#41515=CARTESIAN_POINT('Ctrl Pts',(5.99974507579593,-4.12071884617363,14.));
#41516=CARTESIAN_POINT('Ctrl Pts',(6.01596626965895,-4.09383803111747,14.));
#41517=CARTESIAN_POINT('Ctrl Pts',(6.03200571335301,-4.06685583684996,14.));
#41518=CARTESIAN_POINT('Ctrl Pts',(6.13148189978188,-3.89951301384362,14.));
#41519=CARTESIAN_POINT('Ctrl Pts',(6.22397103273323,-3.72827256414755,14.));
#41520=CARTESIAN_POINT('Ctrl Pts',(6.30936757032185,-3.5536058398909,14.));
#41521=CARTESIAN_POINT('Ctrl Pts',(6.39501944450721,-3.37841686018694,14.));
#41522=CARTESIAN_POINT('Ctrl Pts',(6.47353642951823,-3.19978038055714,14.));
#41523=CARTESIAN_POINT('Ctrl Pts',(6.54476252176001,-3.01815506875983,14.));
#41524=CARTESIAN_POINT('Ctrl Pts',(6.58134872441318,-2.92486088041935,14.));
#41525=CARTESIAN_POINT('Ctrl Pts',(6.61601041067235,-2.83077788216511,14.));
#41526=CARTESIAN_POINT('Ctrl Pts',(6.64872113712823,-2.73596743377932,14.));
#41527=CARTESIAN_POINT('Ctrl Pts',(6.6641565496469,-2.69122864193718,14.));
#41528=CARTESIAN_POINT('Ctrl Pts',(6.67915749473869,-2.64632786691611,14.));
#41529=CARTESIAN_POINT('Ctrl Pts',(6.6937209078782,-2.60127154668905,14.));
#41530=CARTESIAN_POINT('Ctrl Pts',(6.70351950304729,-2.57095663098317,14.));
#41531=CARTESIAN_POINT('Ctrl Pts',(6.71312002789513,-2.54057130140322,14.));
#41532=CARTESIAN_POINT('Ctrl Pts',(6.72252150160785,-2.51011752011723,14.));
#41533=CARTESIAN_POINT('Ctrl Pts',(6.72982180473667,-2.48646996850992,14.));
#41534=CARTESIAN_POINT('Ctrl Pts',(6.73700164922378,-2.46278244924519,14.));
#41535=CARTESIAN_POINT('Ctrl Pts',(6.74405795301005,-2.43906513842396,14.));
#41536=CARTESIAN_POINT('Ctrl Pts',(6.79911253488915,-2.25401831077738,14.));
#41537=CARTESIAN_POINT('Ctrl Pts',(6.84669881313537,-2.06700471360453,14.));
#41538=CARTESIAN_POINT('Ctrl Pts',(6.88668373523586,-1.87847518436181,14.));
#41539=CARTESIAN_POINT('Ctrl Pts',(6.92645168310919,-1.69096869197288,14.));
#41540=CARTESIAN_POINT('Ctrl Pts',(6.95870064560547,-1.50196198674046,14.));
#41541=CARTESIAN_POINT('Ctrl Pts',(6.98324861503862,-1.31189363116468,14.));
#41542=CARTESIAN_POINT('Ctrl Pts',(7.00741036693461,-1.12481565458474,14.));
#41543=CARTESIAN_POINT('Ctrl Pts',(7.02411155235519,-0.936708550057791,
14.));
#41544=CARTESIAN_POINT('Ctrl Pts',(7.03312830125131,-0.747995340106631,
14.));
#41545=CARTESIAN_POINT('Ctrl Pts',(7.03429963262975,-0.723480328444643,
14.));
#41546=CARTESIAN_POINT('Ctrl Pts',(7.03534121362652,-0.698955102669467,
14.));
#41547=CARTESIAN_POINT('Ctrl Pts',(7.03625248964568,-0.674420604634066,
14.));
#41548=CARTESIAN_POINT('Ctrl Pts',(-7.92543898861653,-0.000149382597450273,
13.7673131746348));
#41549=CARTESIAN_POINT('Ctrl Pts',(-7.92557446574483,-0.15883239438947,
13.7720941892239));
#41550=CARTESIAN_POINT('Ctrl Pts',(-7.92090561055472,-0.317507367685049,
13.776875203813));
#41551=CARTESIAN_POINT('Ctrl Pts',(-7.91137809126235,-0.475890009351388,
13.7816562184022));
#41552=CARTESIAN_POINT('Ctrl Pts',(-7.83245902535478,-1.7878170443658,13.8212586787999));
#41553=CARTESIAN_POINT('Ctrl Pts',(-7.42017413564185,-3.07968643136085,
13.8608611391976));
#41554=CARTESIAN_POINT('Ctrl Pts',(-6.72456199968518,-4.19481298313701,
13.9004635995953));
#41555=CARTESIAN_POINT('Ctrl Pts',(-6.14178063209989,-5.12906203268961,
13.9336423997302));
#41556=CARTESIAN_POINT('Ctrl Pts',(-5.36013105826123,-5.93925477959532,
13.9668211998651));
#41557=CARTESIAN_POINT('Ctrl Pts',(-4.44940638321884,-6.55843917088993,
14.));
#41558=CARTESIAN_POINT('',(-4.10246908460462,-5.75649127412218,-9.32299418528667E-16));
#41559=CARTESIAN_POINT('Ctrl Pts',(-4.10246908460462,-5.75649127412218,
-4.85722573273506E-16));
#41560=CARTESIAN_POINT('Ctrl Pts',(-4.26444805314231,-5.65499654616439,
-4.4106029540016E-16));
#41561=CARTESIAN_POINT('Ctrl Pts',(-4.42206063548502,-5.5470406348928,-4.66377136522777E-16));
#41562=CARTESIAN_POINT('Ctrl Pts',(-4.57488596535248,-5.43284881268837,
-3.64291929955129E-16));
#41563=CARTESIAN_POINT('Ctrl Pts',(-4.7279374413068,-5.31848801303912,-2.54051805889774E-16));
#41564=CARTESIAN_POINT('Ctrl Pts',(-4.87618830111391,-5.19787277182883,
-1.22736874955051E-16));
#41565=CARTESIAN_POINT('Ctrl Pts',(-5.01939433701872,-5.07141828023167,
-1.11022302462516E-16));
#41566=CARTESIAN_POINT('Ctrl Pts',(-5.11357307205341,-4.98825611473475,
-1.033182723087E-16));
#41567=CARTESIAN_POINT('Ctrl Pts',(-5.20556947047894,-4.90256748118548,
2.24781300563221E-16));
#41568=CARTESIAN_POINT('Ctrl Pts',(-5.29530739400484,-4.81446023940099,
2.28983498828939E-16));
#41569=CARTESIAN_POINT('Ctrl Pts',(-5.35325244632467,-4.75756814145219,
2.31696917958756E-16));
#41570=CARTESIAN_POINT('Ctrl Pts',(-5.410255722498,-4.69966745324811,-9.24391999260675E-17));
#41571=CARTESIAN_POINT('Ctrl Pts',(-5.46629534973171,-4.64078562778477,
-4.85722573273506E-17));
#41572=CARTESIAN_POINT('Ctrl Pts',(-5.48682578374535,-4.61921393839368,
-3.25013550951246E-17));
#41573=CARTESIAN_POINT('Ctrl Pts',(-5.50722813752232,-4.59750918490477,
-9.10536588563158E-17));
#41574=CARTESIAN_POINT('Ctrl Pts',(-5.52749729586896,-4.57567699269403,
-8.32667268468867E-17));
#41575=CARTESIAN_POINT('Ctrl Pts',(-5.65993255342473,-4.43302913583735,
-3.23882281642257E-17));
#41576=CARTESIAN_POINT('Ctrl Pts',(-5.78644919432292,-4.28519877405637,
-5.70912284577127E-17));
#41577=CARTESIAN_POINT('Ctrl Pts',(-5.90680145533567,-4.13262192737494,
-9.71445146547012E-17));
#41578=CARTESIAN_POINT('Ctrl Pts',(-6.0276504790816,-3.97941530863324,-1.37363123711073E-16));
#41579=CARTESIAN_POINT('Ctrl Pts',(-6.14228463266651,-3.82142243224172,
-4.75715598069395E-16));
#41580=CARTESIAN_POINT('Ctrl Pts',(-6.25042286356285,-3.65904284819727,
-3.19189119579733E-16));
#41581=CARTESIAN_POINT('Ctrl Pts',(-6.35563422902385,-3.50105822408518,
-1.66899181079758E-16));
#41582=CARTESIAN_POINT('Ctrl Pts',(-6.45469683435067,-3.33892050695521,
-5.21246859396646E-16));
#41583=CARTESIAN_POINT('Ctrl Pts',(-6.54731588099908,-3.17296682181485,
-6.66133814775094E-16));
#41584=CARTESIAN_POINT('Ctrl Pts',(-6.56727385003151,-3.13720637481497,
-6.97354708028551E-16));
#41585=CARTESIAN_POINT('Ctrl Pts',(-6.58693247668688,-3.1012686417294,1.04004692438599E-16));
#41586=CARTESIAN_POINT('Ctrl Pts',(-6.60628856479337,-3.06515684386158,
8.32667268468867E-17));
#41587=CARTESIAN_POINT('Ctrl Pts',(-6.6188568578988,-3.04170873504589,6.98011531972333E-17));
#41588=CARTESIAN_POINT('Ctrl Pts',(-6.6312938824366,-3.01819411604075,-7.91234734162241E-17));
#41589=CARTESIAN_POINT('Ctrl Pts',(-6.6435963695148,-2.99461910387611,-8.32667268468867E-17));
#41590=CARTESIAN_POINT('Ctrl Pts',(-6.70027332772065,-2.88601017214828,
-1.02354493412573E-16));
#41591=CARTESIAN_POINT('Ctrl Pts',(-6.75411340828003,-2.77608610999039,
-1.33518598772074E-16));
#41592=CARTESIAN_POINT('Ctrl Pts',(-6.80505784431399,-2.66494979480104,
-1.11022302462516E-16));
#41593=CARTESIAN_POINT('Ctrl Pts',(-6.8859011242357,-2.48858854835737,-7.74867130424257E-17));
#41594=CARTESIAN_POINT('Ctrl Pts',(-6.95945491899237,-2.30917619159457,
3.04971634102744E-16));
#41595=CARTESIAN_POINT('Ctrl Pts',(-7.02573737023362,-2.12720445243301,
2.4980018054066E-16));
#41596=CARTESIAN_POINT('Ctrl Pts',(-7.09286231827722,-1.94291972385284,
1.93927458809757E-16));
#41597=CARTESIAN_POINT('Ctrl Pts',(-7.15253014845298,-1.75600954554244,
2.61861991801936E-16));
#41598=CARTESIAN_POINT('Ctrl Pts',(-7.20471497950316,-1.56695488902645,
4.16333634234434E-16));
#41599=CARTESIAN_POINT('Ctrl Pts',(-7.25719534398338,-1.37682957711156,
5.71680081345093E-16));
#41600=CARTESIAN_POINT('Ctrl Pts',(-7.30210793162369,-1.18453476783516,
-2.26663475651839E-16));
#41601=CARTESIAN_POINT('Ctrl Pts',(-7.33937802283127,-0.990539282908711,
-2.4980018054066E-16));
#41602=CARTESIAN_POINT('Ctrl Pts',(-7.36972363521549,-0.832586576083263,
-2.68638274456075E-16));
#41603=CARTESIAN_POINT('Ctrl Pts',(-7.3950019111505,-0.673505889728574,
2.62252831393826E-16));
#41604=CARTESIAN_POINT('Ctrl Pts',(-7.41514750937589,-0.513545051200431,
3.05311331771918E-16));
#41605=CARTESIAN_POINT('Ctrl Pts',(-7.41978506017856,-0.476721795479128,
3.1522347142427E-16));
#41606=CARTESIAN_POINT('Ctrl Pts',(-7.4241505193075,-0.439851888410535,
-2.15849517642311E-16));
#41607=CARTESIAN_POINT('Ctrl Pts',(-7.4282429147508,-0.402938341593615,
-2.22044604925031E-16));
#41608=CARTESIAN_POINT('Ctrl Pts',(-7.43102427808838,-0.377850349194206,
-2.26255045699889E-16));
#41609=CARTESIAN_POINT('Ctrl Pts',(-7.43367975165298,-0.35273976384182,
6.84940450236123E-16));
#41610=CARTESIAN_POINT('Ctrl Pts',(-7.43620823019086,-0.327615359508083,
6.66133814775094E-16));
#41611=CARTESIAN_POINT('Ctrl Pts',(-7.45623500882372,-0.12861786898675,
5.17176123592382E-16));
#41612=CARTESIAN_POINT('Ctrl Pts',(-7.46825515329086,0.0707954497941199,
5.08633511213826E-16));
#41613=CARTESIAN_POINT('Ctrl Pts',(-7.47226868254779,0.270127329357898,
3.88578058618805E-16));
#41614=CARTESIAN_POINT('Ctrl Pts',(-7.47631137746368,0.470907721003539,
2.6765018273676E-16));
#41615=CARTESIAN_POINT('Ctrl Pts',(-7.47223087939926,0.671606167152592,
-2.90044233826028E-16));
#41616=CARTESIAN_POINT('Ctrl Pts',(-7.45997809674896,0.871732927784226,
-3.88578058618805E-16));
#41617=CARTESIAN_POINT('Ctrl Pts',(-7.45874178840682,0.891925759952658,
-3.98520142229585E-16));
#41618=CARTESIAN_POINT('Ctrl Pts',(-7.45742223668918,0.912112782108578,
-5.92394325853002E-17));
#41619=CARTESIAN_POINT('Ctrl Pts',(-7.45601936233051,0.932293497244242,
-5.55111512312578E-17));
#41620=CARTESIAN_POINT('Ctrl Pts',(-7.44220469443973,1.13102111363738,-1.87972656354744E-17));
#41621=CARTESIAN_POINT('Ctrl Pts',(-7.42031449996691,1.32913694415759,-2.12031727035272E-16));
#41622=CARTESIAN_POINT('Ctrl Pts',(-7.39055416059426,1.52620370719721,-2.22044604925031E-16));
#41623=CARTESIAN_POINT('Ctrl Pts',(-7.36063263652316,1.72433780170694,-2.32111713469992E-16));
#41624=CARTESIAN_POINT('Ctrl Pts',(-7.32275536562233,1.92141211023425,5.3721443045487E-16));
#41625=CARTESIAN_POINT('Ctrl Pts',(-7.27707851263434,2.11697850450149,5.55111512312578E-16));
#41626=CARTESIAN_POINT('Ctrl Pts',(-7.25245833225854,2.22239031786722,5.64758179162703E-16));
#41627=CARTESIAN_POINT('Ctrl Pts',(-7.22557125362165,2.3273639139264,-6.15445996968898E-16));
#41628=CARTESIAN_POINT('Ctrl Pts',(-7.1964356368219,2.43182760644158,-6.10622663543836E-16));
#41629=CARTESIAN_POINT('Ctrl Pts',(-7.18741574955678,2.46416777401931,-6.09129442238959E-16));
#41630=CARTESIAN_POINT('Ctrl Pts',(-7.17818032873551,2.49645906127832,2.62623543107519E-16));
#41631=CARTESIAN_POINT('Ctrl Pts',(-7.1687298384034,2.52869931099089,2.77555756156289E-16));
#41632=CARTESIAN_POINT('Ctrl Pts',(-7.16155733462016,2.55316823322769,2.88888644802346E-16));
#41633=CARTESIAN_POINT('Ctrl Pts',(-7.15426051935625,2.57760900340121,6.20963924433363E-16));
#41634=CARTESIAN_POINT('Ctrl Pts',(-7.14684494823062,2.60200349713766,6.10622663543836E-16));
#41635=CARTESIAN_POINT('Ctrl Pts',(-7.08779443525734,2.7962579037715,5.28274756690613E-16));
#41636=CARTESIAN_POINT('Ctrl Pts',(-7.02114659736257,2.98782550259838,-1.80070095916221E-16));
#41637=CARTESIAN_POINT('Ctrl Pts',(-6.94715442945099,3.17626378280464,-1.66533453693773E-16));
#41638=CARTESIAN_POINT('Ctrl Pts',(-6.87263508283784,3.36604464629625,-1.52900365730218E-16));
#41639=CARTESIAN_POINT('Ctrl Pts',(-6.79066624250823,3.55265212440146,7.72926337156281E-16));
#41640=CARTESIAN_POINT('Ctrl Pts',(-6.70145334111822,3.73563167634114,6.66133814775094E-16));
#41641=CARTESIAN_POINT('Ctrl Pts',(-6.6123241367756,3.91843956198602,5.59441482149727E-16));
#41642=CARTESIAN_POINT('Ctrl Pts',(-6.51596425805218,4.09762701399909,3.57827323897638E-16));
#41643=CARTESIAN_POINT('Ctrl Pts',(-6.41252847447672,4.27272797583501,4.44089209850063E-16));
#41644=CARTESIAN_POINT('Ctrl Pts',(-6.36760697881687,4.34877319756825,4.81552192209496E-16));
#41645=CARTESIAN_POINT('Ctrl Pts',(-6.32135026893501,4.42404743802936,-4.14513171145246E-16));
#41646=CARTESIAN_POINT('Ctrl Pts',(-6.27376821910516,4.49851126261938,-4.44089209850063E-16));
#41647=CARTESIAN_POINT('Ctrl Pts',(-6.18645080840074,4.63515918715393,-4.99268523196803E-16));
#41648=CARTESIAN_POINT('Ctrl Pts',(-6.09467122636726,4.76907872895868,-1.98525553334617E-16));
#41649=CARTESIAN_POINT('Ctrl Pts',(-5.99860552186345,4.90011413024603,-2.22044604925031E-16));
#41650=CARTESIAN_POINT('Ctrl Pts',(-5.95657677614303,4.95744211830925,-2.32334189995837E-16));
#41651=CARTESIAN_POINT('Ctrl Pts',(-5.91372741630838,5.01421790698281,4.04725268970026E-17));
#41652=CARTESIAN_POINT('Ctrl Pts',(-5.8700711905739,5.07042766638301,5.55111512312578E-17));
#41653=CARTESIAN_POINT('Ctrl Pts',(-5.84847106648942,5.09823899815474,6.2951926200114E-17));
#41654=CARTESIAN_POINT('Ctrl Pts',(-5.82667340878159,5.12591175532134,1.17875647828567E-16));
#41655=CARTESIAN_POINT('Ctrl Pts',(-5.80467983186185,5.1534442149457,1.11022302462516E-16));
#41656=CARTESIAN_POINT('Ctrl Pts',(-5.78581483932773,5.17706018460606,1.05143844873007E-16));
#41657=CARTESIAN_POINT('Ctrl Pts',(-5.76680349838768,5.20057552886117,2.33129696379534E-16));
#41658=CARTESIAN_POINT('Ctrl Pts',(-5.74766328194096,5.22396929474179,2.22044604925031E-16));
#41659=CARTESIAN_POINT('Ctrl Pts',(-5.61867202042286,5.38162641324933,1.47339079272257E-16));
#41660=CARTESIAN_POINT('Ctrl Pts',(-5.48369056578089,5.53394270109696,-8.06489650850003E-16));
#41661=CARTESIAN_POINT('Ctrl Pts',(-5.34315344687823,5.68067077831208,-6.66133814775094E-16));
#41662=CARTESIAN_POINT('Ctrl Pts',(-5.20008363720417,5.83004311670153,-5.23248554918668E-16));
#41663=CARTESIAN_POINT('Ctrl Pts',(-5.05125577950163,5.97362456003765,2.85421131474252E-16));
#41664=CARTESIAN_POINT('Ctrl Pts',(-4.8970796282879,6.11113067320816,2.22044604925031E-16));
#41665=CARTESIAN_POINT('Ctrl Pts',(-4.74253899229358,6.248961861853,1.5851825118664E-16));
#41666=CARTESIAN_POINT('Ctrl Pts',(-4.58262427189498,6.38068947566403,-3.93198157072506E-16));
#41667=CARTESIAN_POINT('Ctrl Pts',(-4.41770596513535,6.50599578022417,-3.88578058618805E-16));
#41668=CARTESIAN_POINT('Ctrl Pts',(-4.2543231982024,6.63013536882073,-3.84000977494824E-16));
#41669=CARTESIAN_POINT('Ctrl Pts',(-4.08602906082971,6.74797310968672,-4.57848538427986E-16));
#41670=CARTESIAN_POINT('Ctrl Pts',(-3.91315002787191,6.85916237355816,-5.55111512312578E-16));
#41671=CARTESIAN_POINT('Ctrl Pts',(-3.76372415357097,6.95526745167325,-6.39179572280059E-16));
#41672=CARTESIAN_POINT('Ctrl Pts',(-3.61087228998677,7.04640519188708,2.86820439889053E-17));
#41673=CARTESIAN_POINT('Ctrl Pts',(-3.45478907940187,7.13232482552818,0.));
#41674=CARTESIAN_POINT('Ctrl Pts',(-4.10246908460462,-5.75649127412218,
-4.82469966756049E-16));
#41675=CARTESIAN_POINT('Ctrl Pts',(-3.30199626649145,-6.32576073711656,
0.0331788001348988));
#41676=CARTESIAN_POINT('Ctrl Pts',(-1.28363269872274,-7.20768574705846,
0.105960060667506));
#41677=CARTESIAN_POINT('Ctrl Pts',(2.14497044005655,-7.04780045183455,0.21834378159782));
#41678=CARTESIAN_POINT('Ctrl Pts',(5.24919481691,-5.16895421862038,0.337151162790942));
#41679=CARTESIAN_POINT('Ctrl Pts',(7.07998577213964,-2.03617489938541,0.455958543984065));
#41680=CARTESIAN_POINT('Ctrl Pts',(7.19320815162393,1.59058620557498,0.574765925177186));
#41681=CARTESIAN_POINT('Ctrl Pts',(5.56139171256912,4.83147080423204,0.693573306370309));
#41682=CARTESIAN_POINT('Ctrl Pts',(2.5804088453257,6.9002678057359,0.812380687563431));
#41683=CARTESIAN_POINT('Ctrl Pts',(-1.02656909712053,7.29509087359264,0.931188068756555));
#41684=CARTESIAN_POINT('Ctrl Pts',(-4.3845061645243,5.92016094290675,1.04999544994967));
#41685=CARTESIAN_POINT('Ctrl Pts',(-6.58353186552137,3.22573736676226,1.16387031672212));
#41686=CARTESIAN_POINT('Ctrl Pts',(-7.0679837071718,1.02621179261826,1.23814272309686));
#41687=CARTESIAN_POINT('Ctrl Pts',(-7.06887577069393,-0.000134259091651625,
1.27281266907389));
#41688=CARTESIAN_POINT('Origin',(0.,0.,-2.77281266907387));
#41689=CARTESIAN_POINT('',(4.10219162127161,-5.75636310115763,0.));
#41690=CARTESIAN_POINT('Origin',(0.,0.,0.));
#41691=CARTESIAN_POINT('Ctrl Pts',(4.1021916212716,-5.75636310115763,-1.66533453693773E-15));
#41692=CARTESIAN_POINT('Ctrl Pts',(5.05709396285032,-5.0758653083813,0.0396024603977058));
#41693=CARTESIAN_POINT('Ctrl Pts',(6.62078237616492,-3.2312072264826,0.11880738119312));
#41694=CARTESIAN_POINT('Ctrl Pts',(7.35993086199691,0.321887848378951,0.237614762386243));
#41695=CARTESIAN_POINT('Ctrl Pts',(6.31364411820374,3.79596318205578,0.356422143579365));
#41696=CARTESIAN_POINT('Ctrl Pts',(3.73567782192208,6.34961322753113,0.475229524772488));
#41697=CARTESIAN_POINT('Ctrl Pts',(0.25146363409415,7.3626457790994,0.594036905965609));
#41698=CARTESIAN_POINT('Ctrl Pts',(-3.29375929907944,6.58965400328772,0.712844287158733));
#41699=CARTESIAN_POINT('Ctrl Pts',(-6.03992954092638,4.21798341238717,0.831651668351853));
#41700=CARTESIAN_POINT('Ctrl Pts',(-6.9899282991103,1.70012972441635,0.919766016274316));
#41701=CARTESIAN_POINT('Ctrl Pts',(-7.06879097449385,0.263968838154456,
0.96827790379907));
#41702=CARTESIAN_POINT('Ctrl Pts',(-7.06852116118549,0.000181853424906647,
0.977187330926117));
#41703=CARTESIAN_POINT('Ctrl Pts',(4.59925989935307,-6.4538696437256,-0.494500505560915));
#41704=CARTESIAN_POINT('Ctrl Pts',(5.66986908899888,-5.69091498463918,-0.454898045163208));
#41705=CARTESIAN_POINT('Ctrl Pts',(7.42303180747073,-3.62273711110913,-0.375693124367793));
#41706=CARTESIAN_POINT('Ctrl Pts',(8.25174394586199,0.360891447747451,-0.256885743174671));
#41707=CARTESIAN_POINT('Ctrl Pts',(7.07867717857605,4.25592533320956,-0.138078361981549));
#41708=CARTESIAN_POINT('Ctrl Pts',(4.18833511193785,7.11900471502922,-0.0192709807884262));
#41709=CARTESIAN_POINT('Ctrl Pts',(0.281933833231448,8.25478783325497,0.0995364004046958));
#41710=CARTESIAN_POINT('Ctrl Pts',(-3.69286870555341,7.38813156625243,0.218343781597819));
#41711=CARTESIAN_POINT('Ctrl Pts',(-6.77179622435331,4.7290823432367,0.33715116279094));
#41712=CARTESIAN_POINT('Ctrl Pts',(-8.20791988552602,0.92281499234215,0.455958543984063));
#41713=CARTESIAN_POINT('Ctrl Pts',(-7.65284082860589,-3.10734050142714,
0.574765925177185));
#41714=CARTESIAN_POINT('Ctrl Pts',(-5.24121966776055,-6.38366107966517,
0.693573306370307));
#41715=CARTESIAN_POINT('Ctrl Pts',(-1.55810356768701,-8.11134070632496,
0.81238068756343));
#41716=CARTESIAN_POINT('Ctrl Pts',(2.50300088702735,-7.87124563541711,0.931188068756552));
#41717=CARTESIAN_POINT('Ctrl Pts',(5.95688938266422,-5.72162533208904,1.04999544994967));
#41718=CARTESIAN_POINT('Ctrl Pts',(7.96566506351131,-2.18396555594479,1.1688028311428));
#41719=CARTESIAN_POINT('Ctrl Pts',(8.0420086234621,1.88351347449462,1.28761021233592));
#41720=CARTESIAN_POINT('Ctrl Pts',(6.16739946160646,5.49406133107593,1.40641759352904));
#41721=CARTESIAN_POINT('Ctrl Pts',(2.79660877821874,7.77177618156632,1.52522497472216));
#41722=CARTESIAN_POINT('Ctrl Pts',(-1.2526257813883,8.16409545269238,1.64403235591529));
#41723=CARTESIAN_POINT('Ctrl Pts',(-4.99797933429252,6.57584430815122,1.76283973710841));
#41724=CARTESIAN_POINT('Ctrl Pts',(-7.53084707602691,3.39232488910422,1.88164711830153));
#41725=CARTESIAN_POINT('Ctrl Pts',(-8.23676744172077,-0.614156280905575,
2.00045449949465));
#41726=CARTESIAN_POINT('Ctrl Pts',(-6.94448753724244,-4.4716460803835,2.11926188068778));
#41727=CARTESIAN_POINT('Ctrl Pts',(-3.96750826828504,-7.2443359923163,2.2380692618809));
#41728=CARTESIAN_POINT('Ctrl Pts',(-0.0280305252716536,-8.25958474223567,
2.35687664307402));
#41729=CARTESIAN_POINT('Ctrl Pts',(3.91824728872815,-7.27109785459193,2.47568402426714));
#41730=CARTESIAN_POINT('Ctrl Pts',(6.91397710597332,-4.51867750606856,2.59449140546026));
#41731=CARTESIAN_POINT('Ctrl Pts',(8.23240924307313,-0.670047670383021,
2.71329878665339));
#41732=CARTESIAN_POINT('Ctrl Pts',(7.55369838796778,3.34113251602617,2.83210616784651));
#41733=CARTESIAN_POINT('Ctrl Pts',(5.04249653839076,6.54176998115001,2.95091354903963));
#41734=CARTESIAN_POINT('Ctrl Pts',(1.30800921702632,8.15540542917379,3.06972093023275));
#41735=CARTESIAN_POINT('Ctrl Pts',(-2.74379486597955,7.79057864085904,3.18852831142588));
#41736=CARTESIAN_POINT('Ctrl Pts',(-6.12996747624935,5.53579484501796,3.307335692619));
#41737=CARTESIAN_POINT('Ctrl Pts',(-8.02903938171325,1.9380537745105,3.42614307381212));
#41738=CARTESIAN_POINT('Ctrl Pts',(-7.98030484779208,-2.12984984501333,
3.54495045500524));
#41739=CARTESIAN_POINT('Ctrl Pts',(-5.99558663863968,-5.68106210884581,
3.66375783619837));
#41740=CARTESIAN_POINT('Ctrl Pts',(-2.5563678712721,-7.85407595664345,3.78256521739149));
#41741=CARTESIAN_POINT('Ctrl Pts',(1.50301347898698,-8.12172865269342,3.90137259858461));
#41742=CARTESIAN_POINT('Ctrl Pts',(5.19777096907156,-6.41908893684097,4.02017997977773));
#41743=CARTESIAN_POINT('Ctrl Pts',(7.63157415532434,-3.15920903673424,4.13898736097086));
#41744=CARTESIAN_POINT('Ctrl Pts',(8.21399405950708,0.867079821227378,4.25779474216397));
#41745=CARTESIAN_POINT('Ctrl Pts',(6.80373840668384,4.68301927386732,4.3766021233571));
#41746=CARTESIAN_POINT('Ctrl Pts',(3.74292845335315,7.36288071471193,4.49540950455022));
#41747=CARTESIAN_POINT('Ctrl Pts',(-0.225897988251801,8.25654261327956,
4.61421688574334));
#41748=CARTESIAN_POINT('Ctrl Pts',(-4.13992266152032,7.14720687979774,4.73302426693647));
#41749=CARTESIAN_POINT('Ctrl Pts',(-7.04962195596062,4.30399304182004,4.85183164812958));
#41750=CARTESIAN_POINT('Ctrl Pts',(-8.2491167803214,0.416651137785123,4.97063902932272));
#41751=CARTESIAN_POINT('Ctrl Pts',(-7.44741544408726,-3.57176833363641,
5.08944641051582));
#41752=CARTESIAN_POINT('Ctrl Pts',(-4.83900684573563,-6.69369394078645,
5.20825379170897));
#41753=CARTESIAN_POINT('Ctrl Pts',(-1.05667839891248,-8.19176150698183,
5.32706117290206));
#41754=CARTESIAN_POINT('Ctrl Pts',(2.98199515869051,-7.70254702676615,5.44586855409521));
#41755=CARTESIAN_POINT('Ctrl Pts',(6.29725099517214,-5.34473158631946,5.56467593528831));
#41756=CARTESIAN_POINT('Ctrl Pts',(8.08482394760204,-1.69030990125421,5.68348331648146));
#41757=CARTESIAN_POINT('Ctrl Pts',(7.91105739255604,2.37417285758257,5.80229069767456));
#41758=CARTESIAN_POINT('Ctrl Pts',(5.81810626274495,5.86269266987495,5.92109807886769));
#41759=CARTESIAN_POINT('Ctrl Pts',(2.31371046255249,7.92895136329341,6.0399054600608));
#41760=CARTESIAN_POINT('Ctrl Pts',(-1.75198039718303,8.07168449048177,6.15871284125393));
#41761=CARTESIAN_POINT('Ctrl Pts',(-5.39264921666282,6.25626567946273,6.27752022244705));
#41762=CARTESIAN_POINT('Ctrl Pts',(-7.72508720425954,2.92310682538001,6.39632760364018));
#41763=CARTESIAN_POINT('Ctrl Pts',(-8.18345609268867,-1.11918372264528,
6.51513498483329));
#41764=CARTESIAN_POINT('Ctrl Pts',(-6.6565577883739,-4.88996566818585,6.63394236602643));
#41765=CARTESIAN_POINT('Ctrl Pts',(-3.51481049554077,-7.47446539937364,
6.75274974721954));
#41766=CARTESIAN_POINT('Ctrl Pts',(0.479612963263723,-8.24569567904776,
6.87155712841267));
#41767=CARTESIAN_POINT('Ctrl Pts',(4.35768461784302,-7.01655974088526,6.99036450960579));
#41768=CARTESIAN_POINT('Ctrl Pts',(7.17860288757583,-4.08524006742388,7.10917189079891));
#41769=CARTESIAN_POINT('Ctrl Pts',(8.25802653192982,-0.162860750154332,
7.22797927199203));
#41770=CARTESIAN_POINT('Ctrl Pts',(7.33409255268801,3.79902780387349,7.34678665318516));
#41771=CARTESIAN_POINT('Ctrl Pts',(4.63094290118184,6.83929043629462,7.46559403437828));
#41772=CARTESIAN_POINT('Ctrl Pts',(0.804348716087926,8.22037401636477,7.5844014155714));
#41773=CARTESIAN_POINT('Ctrl Pts',(-3.21737660913659,7.60723429249936,7.70320879676452));
#41774=CARTESIAN_POINT('Ctrl Pts',(-6.45858180246632,5.14861602052904,7.82201617795764));
#41775=CARTESIAN_POINT('Ctrl Pts',(-8.13296603178495,1.44096819945123,7.94082355915076));
#41776=CARTESIAN_POINT('Ctrl Pts',(-7.83433171493839,-2.61625159461166,
8.05963094034389));
#41777=CARTESIAN_POINT('Ctrl Pts',(-5.6351261046702,-6.038781301758,8.17843832153702));
#41778=CARTESIAN_POINT('Ctrl Pts',(-2.0688659326293,-7.99633163261776,8.29724570273012));
#41779=CARTESIAN_POINT('Ctrl Pts',(1.99929119049366,-8.01401026712669,8.41605308392327));
#41780=CARTESIAN_POINT('Ctrl Pts',(5.5824298612325,-6.08752845335585,8.53486046511637));
#41781=CARTESIAN_POINT('Ctrl Pts',(7.81129782607728,-2.68424143815676,8.65366784630951));
#41782=CARTESIAN_POINT('Ctrl Pts',(8.14518240844654,1.37022967386143,8.77247522750261));
#41783=CARTESIAN_POINT('Ctrl Pts',(6.50308481027346,5.09228963987598,8.89128260869575));
#41784=CARTESIAN_POINT('Ctrl Pts',(3.28337003187236,7.57898456653659,9.01008998988886));
#41785=CARTESIAN_POINT('Ctrl Pts',(-0.732874566214402,8.22705419309936,
9.12889737108199));
#41786=CARTESIAN_POINT('Ctrl Pts',(-4.57132731007446,6.87927993689491,9.24770475227511));
#41787=CARTESIAN_POINT('Ctrl Pts',(-7.30079797677848,3.86262536732011,9.36651213346823));
#41788=CARTESIAN_POINT('Ctrl Pts',(-8.25913007562251,-0.09108358768139,
9.48531951466136));
#41789=CARTESIAN_POINT('Ctrl Pts',(-7.2138368364646,-4.02269610123163,9.60412689585447));
#41790=CARTESIAN_POINT('Ctrl Pts',(-4.41850138494165,-6.97842183715385,
9.7229342770476));
#41791=CARTESIAN_POINT('Ctrl Pts',(-0.551258692607032,-8.24121591027825,
9.84174165824072));
#41792=CARTESIAN_POINT('Ctrl Pts',(3.44971671421322,-7.50473053598029,9.96054903943385));
#41793=CARTESIAN_POINT('Ctrl Pts',(6.61380739416247,-4.94763353320742,10.079356420627));
#41794=CARTESIAN_POINT('Ctrl Pts',(8.17342012615973,-1.19026436865481,10.1981638018201));
#41795=CARTESIAN_POINT('Ctrl Pts',(7.75020034274994,2.8558572221355,10.3169711830132));
#41796=CARTESIAN_POINT('Ctrl Pts',(5.44681913324314,6.20916155014182,10.4357785642063));
#41797=CARTESIAN_POINT('Ctrl Pts',(1.82206572993403,8.05615307089917,10.5545859453995));
#41798=CARTESIAN_POINT('Ctrl Pts',(-2.24471207915242,7.94876050134495,10.6733933265926));
#41799=CARTESIAN_POINT('Ctrl Pts',(-5.76693350554978,5.91303676367643,10.7922007077857));
#41800=CARTESIAN_POINT('Ctrl Pts',(-7.89012452694981,2.4428386715046,10.9110080889788));
#41801=CARTESIAN_POINT('Ctrl Pts',(-8.09920918644618,-1.61998036434483,
11.029815470172));
#41802=CARTESIAN_POINT('Ctrl Pts',(-6.34346454837397,-5.28979993459502,
11.148622851365));
#41803=CARTESIAN_POINT('Ctrl Pts',(-3.04882584022707,-7.67633941566181,
11.2674302325582));
#41804=CARTESIAN_POINT('Ctrl Pts',(0.985443392390751,-8.20063577678695,
11.3862376137513));
#41805=CARTESIAN_POINT('Ctrl Pts',(4.78064878394765,-6.73549723709446,11.5050449949444));
#41806=CARTESIAN_POINT('Ctrl Pts',(7.4160917151457,-3.63635937556868,11.6238523761376));
#41807=CARTESIAN_POINT('Ctrl Pts',(8.25242636618214,0.344941823793669,11.7426597573307));
#41808=CARTESIAN_POINT('Ctrl Pts',(7.08676197563969,4.24256179795868,11.8614671385238));
#41809=CARTESIAN_POINT('Ctrl Pts',(4.20188310742518,7.11095661822702,11.9802745197169));
#41810=CARTESIAN_POINT('Ctrl Pts',(0.297647586663742,8.25426749886389,12.09908190091));
#41811=CARTESIAN_POINT('Ctrl Pts',(-3.67879587591356,7.39513262976418,12.2178892821032));
#41812=CARTESIAN_POINT('Ctrl Pts',(-6.76278097843589,4.74197415548668,12.3366966632963));
#41813=CARTESIAN_POINT('Ctrl Pts',(-8.20614810557995,0.938435308045864,
12.4555040444894));
#41814=CARTESIAN_POINT('Ctrl Pts',(-7.65874257797369,-3.09276307173143,
12.5743114256825));
#41815=CARTESIAN_POINT('Ctrl Pts',(-5.25336379582813,-6.37367269401289,
12.6931188068757));
#41816=CARTESIAN_POINT('Ctrl Pts',(-1.573542283851,-8.10835846930099,12.8119261880688));
#41817=CARTESIAN_POINT('Ctrl Pts',(2.48800937090492,-7.87599816595178,12.9307335692619));
#41818=CARTESIAN_POINT('Ctrl Pts',(5.94598906728439,-5.73295302344607,13.049540950455));
#41819=CARTESIAN_POINT('Ctrl Pts',(7.96148627945122,-2.19913167759206,13.1683483316481));
#41820=CARTESIAN_POINT('Ctrl Pts',(8.04559263830003,1.86820941418339,13.2871557128413));
#41821=CARTESIAN_POINT('Ctrl Pts',(6.17782291561185,5.48229084249603,13.4059630940344));
#41822=CARTESIAN_POINT('Ctrl Pts',(2.81144855713387,7.76647514340256,13.5247704752275));
#41823=CARTESIAN_POINT('Ctrl Pts',(-1.23717676555208,8.16639239144963,13.6435778564206));
#41824=CARTESIAN_POINT('Ctrl Pts',(-4.98526003051727,6.5854918732965,13.7623852376137));
#41825=CARTESIAN_POINT('Ctrl Pts',(-7.52478211903276,3.40635867929589,13.8811926188069));
#41826=CARTESIAN_POINT('Ctrl Pts',(-7.9994255260722,0.73696682530501,13.9603975396023));
#41827=CARTESIAN_POINT('Ctrl Pts',(-7.90416902665075,-0.574227305285002,
14.));
#41828=CARTESIAN_POINT('Ctrl Pts',(4.43357047332591,-6.22136746286961,-0.329667003707277));
#41829=CARTESIAN_POINT('Ctrl Pts',(5.46561071361603,-5.48589842588655,-0.29006454330957));
#41830=CARTESIAN_POINT('Ctrl Pts',(7.1556153303688,-3.49222714956696,-0.210859622514155));
#41831=CARTESIAN_POINT('Ctrl Pts',(7.95447291790696,0.347890247957953,-0.0920522413210329));
#41832=CARTESIAN_POINT('Ctrl Pts',(6.82366615845194,4.10260461615829,0.0267551398720893));
#41833=CARTESIAN_POINT('Ctrl Pts',(4.03744934859926,6.8625408858632,0.145562521065212));
#41834=CARTESIAN_POINT('Ctrl Pts',(0.271777100185677,7.95740714853644,0.264369902258334));
#41835=CARTESIAN_POINT('Ctrl Pts',(-3.55983223672874,7.12197237859753,0.383177283451457));
#41836=CARTESIAN_POINT('Ctrl Pts',(-6.52784066321101,4.55871603295351,0.501984664644578));
#41837=CARTESIAN_POINT('Ctrl Pts',(-7.91222762971306,0.889570363911394,
0.620792045837701));
#41838=CARTESIAN_POINT('Ctrl Pts',(-7.37714542714633,-2.99539782468805,
0.739599427030823));
#41839=CARTESIAN_POINT('Ctrl Pts',(-5.05240348919327,-6.15368817894034,
0.858406808223945));
#41840=CARTESIAN_POINT('Ctrl Pts',(-1.50197251802458,-7.81912773829268,
0.977214189417068));
#41841=CARTESIAN_POINT('Ctrl Pts',(2.41282968787957,-7.58768214911912,1.09602157061019));
#41842=CARTESIAN_POINT('Ctrl Pts',(5.74229103329506,-5.51550242580367,1.21482895180331));
#41843=CARTESIAN_POINT('Ctrl Pts',(7.67870009497725,-2.10528768008078,1.33363633299643));
#41844=CARTESIAN_POINT('Ctrl Pts',(7.75229336011844,1.81565945594976,1.45244371418956));
#41845=CARTESIAN_POINT('Ctrl Pts',(5.94521743683818,5.29613647176714,1.57125109538268));
#41846=CARTESIAN_POINT('Ctrl Pts',(2.69586028532517,7.4917961058771,1.6900584765758));
#41847=CARTESIAN_POINT('Ctrl Pts',(-1.20749964125124,7.8699819824408,1.80886585776893));
#41848=CARTESIAN_POINT('Ctrl Pts',(-4.81792594628742,6.33894796115095,1.92767323896204));
#41849=CARTESIAN_POINT('Ctrl Pts',(-7.25954652836689,3.27011558237369,2.04648062015517));
#41850=CARTESIAN_POINT('Ctrl Pts',(-7.94003594587077,-0.592031155580847,
2.16528800134829));
#41851=CARTESIAN_POINT('Ctrl Pts',(-6.69431073069572,-4.31055397237727,
2.28409538254141));
#41852=CARTESIAN_POINT('Ctrl Pts',(-3.82457784423514,-6.9833570742335,2.40290276373453));
#41853=CARTESIAN_POINT('Ctrl Pts',(-0.0270207189669029,-7.96203124773619,
2.52171014492766));
#41854=CARTESIAN_POINT('Ctrl Pts',(3.77709150312162,-7.00915483408896,2.64051752612078));
#41855=CARTESIAN_POINT('Ctrl Pts',(6.66489944493164,-4.3558910798247,2.7593249073139));
#41856=CARTESIAN_POINT('Ctrl Pts',(7.93583475236053,-0.64590904452883,2.87813228850702));
#41857=CARTESIAN_POINT('Ctrl Pts',(7.28157461638861,3.22076742664758,2.99693966970015));
#41858=CARTESIAN_POINT('Ctrl Pts',(4.86083940757555,6.30610116984171,3.11574705089327));
#41859=CARTESIAN_POINT('Ctrl Pts',(1.26088787551702,7.86160501907548,3.23455443208639));
#41860=CARTESIAN_POINT('Ctrl Pts',(-2.64494900676982,7.50992120212525,3.35336181327951));
#41861=CARTESIAN_POINT('Ctrl Pts',(-5.90913394760972,5.33636652599553,3.47216919447264));
#41862=CARTESIAN_POINT('Ctrl Pts',(-7.73979133837202,1.86823492875368,3.59097657566576));
#41863=CARTESIAN_POINT('Ctrl Pts',(-7.69281247756563,-2.05312150043904,
3.70978395685888));
#41864=CARTESIAN_POINT('Ctrl Pts',(-5.77959421146849,-5.47640050227478,
3.828591338052));
#41865=CARTESIAN_POINT('Ctrl Pts',(-2.46427411389061,-7.57113101208551,
3.94739871924512));
#41866=CARTESIAN_POINT('Ctrl Pts',(1.44886706280393,-7.8291414564355,4.06620610043825));
#41867=CARTESIAN_POINT('Ctrl Pts',(5.01052004015424,-6.18783973917938,4.18501348163137));
#41868=CARTESIAN_POINT('Ctrl Pts',(7.3566448908013,-3.04539778373894,4.30382086282449));
#41869=CARTESIAN_POINT('Ctrl Pts',(7.91808298013935,0.835843065522612,4.42262824401762));
#41870=CARTESIAN_POINT('Ctrl Pts',(6.55863212086575,4.51431239655639,4.54143562521073));
#41871=CARTESIAN_POINT('Ctrl Pts',(3.60808857027019,7.09763119495797,4.66024300640386));
#41872=CARTESIAN_POINT('Ctrl Pts',(-0.21775995977915,7.95909871219548,4.77905038759697));
#41873=CARTESIAN_POINT('Ctrl Pts',(-3.99078096816209,6.88972706097348,4.8978577687901));
#41874=CARTESIAN_POINT('Ctrl Pts',(-6.79565765710552,4.14894067419358,5.01666514998322));
#41875=CARTESIAN_POINT('Ctrl Pts',(-7.95194039662654,0.401641181969633,
5.13547253117635));
#41876=CARTESIAN_POINT('Ctrl Pts',(-7.1791205407072,-3.44309453436157,5.25427991236947));
#41877=CARTESIAN_POINT('Ctrl Pts',(-4.66468047924256,-6.4525520328881,5.3730872935626));
#41878=CARTESIAN_POINT('Ctrl Pts',(-1.01861130958887,-7.89665136057889,
5.49189467475571));
#41879=CARTESIAN_POINT('Ctrl Pts',(2.87456807757934,-7.42506094775773,5.61070205594884));
#41880=CARTESIAN_POINT('Ctrl Pts',(6.07039103818519,-5.15218636639589,5.72950943714195));
#41881=CARTESIAN_POINT('Ctrl Pts',(7.79356625207644,-1.62941608714592,5.84831681833509));
#41882=CARTESIAN_POINT('Ctrl Pts',(7.62605967828794,2.28864271867535,5.9671241995282));
#41883=CARTESIAN_POINT('Ctrl Pts',(5.60850760810599,5.65148777937031,6.08593158072133));
#41884=CARTESIAN_POINT('Ctrl Pts',(2.23035849573119,7.64330901449592,6.20473896191444));
#41885=CARTESIAN_POINT('Ctrl Pts',(-1.68886488886813,7.78090014700762,6.32354634310758));
#41886=CARTESIAN_POINT('Ctrl Pts',(-5.19837775276918,6.03088222817104,6.44235372430068));
#41887=CARTESIAN_POINT('Ctrl Pts',(-7.44678911002407,2.81780121040889,6.56116110549382));
#41888=CARTESIAN_POINT('Ctrl Pts',(-7.88864515080064,-1.07886486424589,
6.67996848668693));
#41889=CARTESIAN_POINT('Ctrl Pts',(-6.41675371915234,-4.71380349805753,
6.79877586788007));
#41890=CARTESIAN_POINT('Ctrl Pts',(-3.38818861585914,-7.20519601495458,
6.91758324907317));
#41891=CARTESIAN_POINT('Ctrl Pts',(0.462334792789065,-7.94864254133568,
7.0363906302663));
#41892=CARTESIAN_POINT('Ctrl Pts',(4.2006979984873,-6.76378651615052,7.15519801145943));
#41893=CARTESIAN_POINT('Ctrl Pts',(6.9199920201433,-3.93806832745547,7.27400539265254));
#41894=CARTESIAN_POINT('Ctrl Pts',(7.96052917232528,-0.156993653098285,
7.39281277384567));
#41895=CARTESIAN_POINT('Ctrl Pts',(7.06988013328202,3.66216692841534,7.51162015503879));
#41896=CARTESIAN_POINT('Ctrl Pts',(4.4641120875178,6.59290338019847,7.63042753623192));
#41897=CARTESIAN_POINT('Ctrl Pts',(0.775371863287522,7.92423309754179,7.74923491742504));
#41898=CARTESIAN_POINT('Ctrl Pts',(-3.10146985558348,7.33318187729323,7.86804229861817));
#41899=CARTESIAN_POINT('Ctrl Pts',(-6.22590986497684,4.96313591026265,7.98684967981127));
#41900=CARTESIAN_POINT('Ctrl Pts',(-7.83997400628658,1.38905697914291,8.10565706100441));
#41901=CARTESIAN_POINT('Ctrl Pts',(-7.55209806135921,-2.52200051192882,
8.22446444219752));
#41902=CARTESIAN_POINT('Ctrl Pts',(-5.43211935351772,-5.82123277662844,
8.34327182339065));
#41903=CARTESIAN_POINT('Ctrl Pts',(-1.99433454792699,-7.70826189367614,
8.46207920458377));
#41904=CARTESIAN_POINT('Ctrl Pts',(1.92726625233771,-7.72530365119423,8.58088658577689));
#41905=CARTESIAN_POINT('Ctrl Pts',(5.38132150471746,-5.86822380055671,8.69969396697001));
#41906=CARTESIAN_POINT('Ctrl Pts',(7.52989397379399,-2.58754100527426,8.81850134816314));
#41907=CARTESIAN_POINT('Ctrl Pts',(7.85175028508863,1.32086682567376,8.93730872935625));
#41908=CARTESIAN_POINT('Ctrl Pts',(6.2688096413986,4.90883870079905,9.05611611054938));
#41909=CARTESIAN_POINT('Ctrl Pts',(3.16508584965159,7.30594985439198,9.17492349174251));
#41910=CARTESIAN_POINT('Ctrl Pts',(-0.706472586573508,7.93067261932902,
9.29373087293562));
#41911=CARTESIAN_POINT('Ctrl Pts',(-4.40664416218472,6.63145224957837,9.41253825412875));
#41912=CARTESIAN_POINT('Ctrl Pts',(-7.03778500234691,3.72347337459204,9.53134563532187));
#41913=CARTESIAN_POINT('Ctrl Pts',(-7.96159296059536,-0.0878022798854391,
9.65015301651499));
#41914=CARTESIAN_POINT('Ctrl Pts',(-6.95395665768722,-3.87777752244279,
9.76896039770813));
#41915=CARTESIAN_POINT('Ctrl Pts',(-4.25932382716235,-6.72702253942422,
9.88776777890122));
#41916=CARTESIAN_POINT('Ctrl Pts',(-0.531399467781868,-7.94432415729598,
10.0065751600944));
#41917=CARTESIAN_POINT('Ctrl Pts',(3.32543985340467,-7.23437084285444,10.1253825412875));
#41918=CARTESIAN_POINT('Ctrl Pts',(6.37554341800685,-4.76939386459785,10.2441899224806));
#41919=CARTESIAN_POINT('Ctrl Pts',(7.87897073234035,-1.14738481316572,10.3629973036737));
#41920=CARTESIAN_POINT('Ctrl Pts',(7.47099754175875,2.75297429003208,10.4818046848669));
#41921=CARTESIAN_POINT('Ctrl Pts',(5.25059618528844,5.98547503625344,10.60061206606));
#41922=CARTESIAN_POINT('Ctrl Pts',(1.75642538092503,7.76592825049012,10.7194194472531));
#41923=CARTESIAN_POINT('Ctrl Pts',(-2.16384579541766,7.66240452366244,10.8382268284462));
#41924=CARTESIAN_POINT('Ctrl Pts',(-5.55917836159592,5.70001821528151,10.9570342096394));
#41925=CARTESIAN_POINT('Ctrl Pts',(-7.60588092411773,2.35483483040497,11.0758415908324));
#41926=CARTESIAN_POINT('Ctrl Pts',(-7.80743325928778,-1.56162018844322,
11.1946489720256));
#41927=CARTESIAN_POINT('Ctrl Pts',(-6.1149397371991,-5.09923364042129,11.3134563532187));
#41928=CARTESIAN_POINT('Ctrl Pts',(-2.93899116800185,-7.39979747204398,
11.4322637344118));
#41929=CARTESIAN_POINT('Ctrl Pts',(0.949942561030821,-7.90520593271468,
11.5510711156049));
#41930=CARTESIAN_POINT('Ctrl Pts',(4.60842478043762,-6.49284935555622,11.6698784967981));
#41931=CARTESIAN_POINT('Ctrl Pts',(7.14892525651175,-3.50535866872642,11.7886858779912));
#41932=CARTESIAN_POINT('Ctrl Pts',(7.95513075387362,0.33251521298068,11.9074932591843));
#41933=CARTESIAN_POINT('Ctrl Pts',(6.83145969878857,4.08972250542654,12.0263006403774));
#41934=CARTESIAN_POINT('Ctrl Pts',(4.05050927434379,6.85478272365244,12.1451080215706));
#41935=CARTESIAN_POINT('Ctrl Pts',(0.286924761932817,7.9569055593149,12.2639154027637));
#41936=CARTESIAN_POINT('Ctrl Pts',(-3.54626638410621,7.12872122713987,12.3827227839568));
#41937=CARTESIAN_POINT('Ctrl Pts',(-6.51915019366069,4.57114341461708,12.5015301651499));
#41938=CARTESIAN_POINT('Ctrl Pts',(-7.91051967855875,0.904627954046215,
12.620337546343));
#41939=CARTESIAN_POINT('Ctrl Pts',(-7.38283456459684,-2.98134555034603,
12.7391449275362));
#41940=CARTESIAN_POINT('Ctrl Pts',(-5.06411012217399,-6.14405962724437,
12.8579523087293));
#41941=CARTESIAN_POINT('Ctrl Pts',(-1.51685505078607,-7.81625293706308,
12.9767596899224));
#41942=CARTESIAN_POINT('Ctrl Pts',(2.39837824467233,-7.59226346861687,13.0955670711156));
#41943=CARTESIAN_POINT('Ctrl Pts',(5.73178340435573,-5.52642203439951,13.2143744523086));
#41944=CARTESIAN_POINT('Ctrl Pts',(7.67467185260159,-2.1199074386075,13.3331818335018));
#41945=CARTESIAN_POINT('Ctrl Pts',(7.75574825997389,1.80090672803206,13.4519892146949));
#41946=CARTESIAN_POINT('Ctrl Pts',(5.9552653834469,5.28479001782315,13.570796595888));
#41947=CARTESIAN_POINT('Ctrl Pts',(2.71016545769389,7.48668603886737,13.6896039770812));
#41948=CARTESIAN_POINT('Ctrl Pts',(-1.19260717986564,7.87219617343589,13.8084113582743));
#41949=CARTESIAN_POINT('Ctrl Pts',(-4.80566485843997,6.34824797047931,13.9272187394674));
#41950=CARTESIAN_POINT('Ctrl Pts',(-7.25370006288338,3.28364380195341,14.0460261206605));
#41951=CARTESIAN_POINT('Ctrl Pts',(-7.71124432888689,0.710417421062149,
14.1252310414559));
#41952=CARTESIAN_POINT('Ctrl Pts',(-7.61941946739412,-0.553540630753928,
14.1648335018536));
#41953=CARTESIAN_POINT('Ctrl Pts',(4.26788104729875,-5.98886528201362,-0.16483350185364));
#41954=CARTESIAN_POINT('Ctrl Pts',(5.26135233823317,-5.28088186713393,-0.125231041455932));
#41955=CARTESIAN_POINT('Ctrl Pts',(6.88819885326686,-3.36171718802478,-0.0460261206605175));
#41956=CARTESIAN_POINT('Ctrl Pts',(7.65720188995193,0.334889048168454,0.0727812605326049));
#41957=CARTESIAN_POINT('Ctrl Pts',(6.56865513832785,3.94928389910703,0.191588641725727));
#41958=CARTESIAN_POINT('Ctrl Pts',(3.88656358526067,6.60607705669717,0.310396022918849));
#41959=CARTESIAN_POINT('Ctrl Pts',(0.261620367139915,7.66002646381791,0.429203404111972));
#41960=CARTESIAN_POINT('Ctrl Pts',(-3.42679576790409,6.85581319094263,0.548010785305094));
#41961=CARTESIAN_POINT('Ctrl Pts',(-6.28388510206869,4.38834972267034,0.666818166498216));
#41962=CARTESIAN_POINT('Ctrl Pts',(-7.61653537390012,0.856325735480628,
0.785625547691338));
#41963=CARTESIAN_POINT('Ctrl Pts',(-7.10145002568676,-2.88345514794895,
0.904432928884462));
#41964=CARTESIAN_POINT('Ctrl Pts',(-4.86358731062599,-5.9237152782155,1.02324031007758));
#41965=CARTESIAN_POINT('Ctrl Pts',(-1.44584146836215,-7.52691477026041,
1.14204769127071));
#41966=CARTESIAN_POINT('Ctrl Pts',(2.32265848873178,-7.30411866282113,1.26085507246383));
#41967=CARTESIAN_POINT('Ctrl Pts',(5.5276926839259,-5.30937951951831,1.37966245365695));
#41968=CARTESIAN_POINT('Ctrl Pts',(7.39173512644319,-2.02660980421676,1.49846983485007));
#41969=CARTESIAN_POINT('Ctrl Pts',(7.46257809677478,1.74780543740488,1.6172772160432));
#41970=CARTESIAN_POINT('Ctrl Pts',(5.72303541206989,5.09821161245836,1.73608459723632));
#41971=CARTESIAN_POINT('Ctrl Pts',(2.59511179243159,7.21181603018786,1.85489197842944));
#41972=CARTESIAN_POINT('Ctrl Pts',(-1.16237350111417,7.57586851218925,1.97369935962256));
#41973=CARTESIAN_POINT('Ctrl Pts',(-4.63787255828232,6.10205161415066,2.09250674081568));
#41974=CARTESIAN_POINT('Ctrl Pts',(-6.98824598070687,3.14790627564318,2.21131412200881));
#41975=CARTESIAN_POINT('Ctrl Pts',(-7.64330445002077,-0.569906030256128,
2.33012150320193));
#41976=CARTESIAN_POINT('Ctrl Pts',(-6.44413392414899,-4.14946186437103,
2.44892888439505));
#41977=CARTESIAN_POINT('Ctrl Pts',(-3.68164742018524,-6.72237815615069,
2.56773626558817));
#41978=CARTESIAN_POINT('Ctrl Pts',(-0.0260109126621464,-7.66447775323672,
2.6865436467813));
#41979=CARTESIAN_POINT('Ctrl Pts',(3.63593571751508,-6.74721181358599,2.80535102797442));
#41980=CARTESIAN_POINT('Ctrl Pts',(6.41582178388996,-4.19310465358082,2.92415840916754));
#41981=CARTESIAN_POINT('Ctrl Pts',(7.63926026164792,-0.62177041867464,3.04296579036066));
#41982=CARTESIAN_POINT('Ctrl Pts',(7.00945084480946,3.10040233726899,3.16177317155378));
#41983=CARTESIAN_POINT('Ctrl Pts',(4.67918227676032,6.0704323585334,3.28058055274691));
#41984=CARTESIAN_POINT('Ctrl Pts',(1.21376653400774,7.56780460897718,3.39938793394003));
#41985=CARTESIAN_POINT('Ctrl Pts',(-2.5461031475601,7.22926376339145,3.51819531513315));
#41986=CARTESIAN_POINT('Ctrl Pts',(-5.68830041897008,5.13693820697311,3.63700269632627));
#41987=CARTESIAN_POINT('Ctrl Pts',(-7.45054329503082,1.79841608299685,3.75581007751939));
#41988=CARTESIAN_POINT('Ctrl Pts',(-7.40532010733917,-1.97639315586476,
3.87461745871252));
#41989=CARTESIAN_POINT('Ctrl Pts',(-5.56360178429729,-5.27173889570375,
3.99342483990564));
#41990=CARTESIAN_POINT('Ctrl Pts',(-2.37218035650913,-7.28818606752757,
4.11223222109876));
#41991=CARTESIAN_POINT('Ctrl Pts',(1.39472064662088,-7.53655426017759,4.23103960229189));
#41992=CARTESIAN_POINT('Ctrl Pts',(4.82326911123691,-5.95659054151778,4.34984698348501));
#41993=CARTESIAN_POINT('Ctrl Pts',(7.08171562627826,-2.93158653074365,4.46865436467813));
#41994=CARTESIAN_POINT('Ctrl Pts',(7.62217190077163,0.80460630981784,4.58746174587126));
#41995=CARTESIAN_POINT('Ctrl Pts',(6.31352583504767,4.34560551924548,4.70626912706437));
#41996=CARTESIAN_POINT('Ctrl Pts',(3.47324868718724,6.832381675204,4.8250765082575));
#41997=CARTESIAN_POINT('Ctrl Pts',(-0.209621931306498,7.66165481111141,
4.94388388945061));
#41998=CARTESIAN_POINT('Ctrl Pts',(-3.84163927480386,6.63224724214921,5.06269127064374));
#41999=CARTESIAN_POINT('Ctrl Pts',(-6.54169335825042,3.99388830656712,5.18149865183686));
#42000=CARTESIAN_POINT('Ctrl Pts',(-7.65476401293167,0.38663122615414,5.30030603302999));
#42001=CARTESIAN_POINT('Ctrl Pts',(-6.91082563732715,-3.31442073508673,
5.41911341422311));
#42002=CARTESIAN_POINT('Ctrl Pts',(-4.49035411274948,-6.21141012498974,
5.53792079541623));
#42003=CARTESIAN_POINT('Ctrl Pts',(-0.980544220265259,-7.60154121417596,
5.65672817660935));
#42004=CARTESIAN_POINT('Ctrl Pts',(2.76714099646817,-7.14757486874929,5.77553555780248));
#42005=CARTESIAN_POINT('Ctrl Pts',(5.84353108119824,-4.95964114647233,5.89434293899559));
#42006=CARTESIAN_POINT('Ctrl Pts',(7.50230855655086,-1.56852227303763,6.01315032018873));
#42007=CARTESIAN_POINT('Ctrl Pts',(7.34106196401981,2.20311257976813,6.13195770138183));
#42008=CARTESIAN_POINT('Ctrl Pts',(5.39890895346704,5.44028288886567,6.25076508257497));
#42009=CARTESIAN_POINT('Ctrl Pts',(2.14700652890988,7.35766666569841,6.36957246376809));
#42010=CARTESIAN_POINT('Ctrl Pts',(-1.62574938055321,7.49011580353348,6.48837984496121));
#42011=CARTESIAN_POINT('Ctrl Pts',(-5.00410628887554,5.80549877687935,6.60718722615433));
#42012=CARTESIAN_POINT('Ctrl Pts',(-7.1684910157886,2.71249559543777,6.72599460734745));
#42013=CARTESIAN_POINT('Ctrl Pts',(-7.59383420891262,-1.03854600584651,
6.84480198854057));
#42014=CARTESIAN_POINT('Ctrl Pts',(-6.17694964993078,-4.5376413279292,6.96360936973371));
#42015=CARTESIAN_POINT('Ctrl Pts',(-3.2615667361775,-6.93592663053551,7.08241675092681));
#42016=CARTESIAN_POINT('Ctrl Pts',(0.445056622314409,-7.65158940362362,
7.20122413211994));
#42017=CARTESIAN_POINT('Ctrl Pts',(4.04371137913158,-6.51101329141579,7.32003151331306));
#42018=CARTESIAN_POINT('Ctrl Pts',(6.66138115271077,-3.79089658748706,7.43883889450619));
#42019=CARTESIAN_POINT('Ctrl Pts',(7.66303181272074,-0.151126556042241,
7.55764627569931));
#42020=CARTESIAN_POINT('Ctrl Pts',(6.80566771387603,3.52530605295721,7.67645365689243));
#42021=CARTESIAN_POINT('Ctrl Pts',(4.29728127385376,6.34651632410231,7.79526103808556));
#42022=CARTESIAN_POINT('Ctrl Pts',(0.746395010487117,7.62809217871881,7.91406841927867));
#42023=CARTESIAN_POINT('Ctrl Pts',(-2.98556310203037,7.0591294620871,8.03287580047181));
#42024=CARTESIAN_POINT('Ctrl Pts',(-5.99323792748737,4.77765579999626,8.15168318166491));
#42025=CARTESIAN_POINT('Ctrl Pts',(-7.54698198078821,1.33714575883459,8.27049056285805));
#42026=CARTESIAN_POINT('Ctrl Pts',(-7.26986440778004,-2.42774942924598,
8.38929794405116));
#42027=CARTESIAN_POINT('Ctrl Pts',(-5.22911260236524,-5.60368425149886,
8.50810532524429));
#42028=CARTESIAN_POINT('Ctrl Pts',(-1.91980316322469,-7.42019215473452,
8.6269127064374));
#42029=CARTESIAN_POINT('Ctrl Pts',(1.85524131418177,-7.43659703526178,8.74572008763054));
#42030=CARTESIAN_POINT('Ctrl Pts',(5.1802131482024,-5.64891914775757,8.86452746882365));
#42031=CARTESIAN_POINT('Ctrl Pts',(7.2484901215107,-2.49084057239175,8.98333485001678));
#42032=CARTESIAN_POINT('Ctrl Pts',(7.55831816173071,1.27150397748608,9.10214223120989));
#42033=CARTESIAN_POINT('Ctrl Pts',(6.03453447252376,4.72538776172215,9.22094961240303));
#42034=CARTESIAN_POINT('Ctrl Pts',(3.04680166743081,7.03291514224736,9.33975699359614));
#42035=CARTESIAN_POINT('Ctrl Pts',(-0.68007060693261,7.63429104555869,9.45856437478927));
#42036=CARTESIAN_POINT('Ctrl Pts',(-4.24196101429499,6.38362456226184,9.57737175598239));
#42037=CARTESIAN_POINT('Ctrl Pts',(-6.77477202791534,3.58432138186396,9.69617913717551));
#42038=CARTESIAN_POINT('Ctrl Pts',(-7.6640558455682,-0.084520972089485,
9.81498651836863));
#42039=CARTESIAN_POINT('Ctrl Pts',(-6.69407647890986,-3.73285894365395,
9.93379389956175));
#42040=CARTESIAN_POINT('Ctrl Pts',(-4.10014626938305,-6.47562324169458,
10.0526012807549));
#42041=CARTESIAN_POINT('Ctrl Pts',(-0.511540242956711,-7.64743240431371,
10.171408661948));
#42042=CARTESIAN_POINT('Ctrl Pts',(3.20116299259612,-6.96401114972859,10.2902160431411));
#42043=CARTESIAN_POINT('Ctrl Pts',(6.13727944185122,-4.59115419598828,10.4090234243342));
#42044=CARTESIAN_POINT('Ctrl Pts',(7.58452133852098,-1.10450525767663,10.5278308055274));
#42045=CARTESIAN_POINT('Ctrl Pts',(7.19179474076756,2.65009135792866,10.6466381867205));
#42046=CARTESIAN_POINT('Ctrl Pts',(5.05437323733374,5.76178852236506,10.7654455679136));
#42047=CARTESIAN_POINT('Ctrl Pts',(1.69078503191604,7.47570343008108,10.8842529491067));
#42048=CARTESIAN_POINT('Ctrl Pts',(-2.0829795116829,7.3760485459799,11.0030603302999));
#42049=CARTESIAN_POINT('Ctrl Pts',(-5.35142321764206,5.4869996668866,11.121867711493));
#42050=CARTESIAN_POINT('Ctrl Pts',(-7.32163732128566,2.26683098930532,11.2406750926861));
#42051=CARTESIAN_POINT('Ctrl Pts',(-7.51565733212937,-1.5032600125416,11.3594824738792));
#42052=CARTESIAN_POINT('Ctrl Pts',(-5.88641492602424,-4.90866734624756,
11.4782898550723));
#42053=CARTESIAN_POINT('Ctrl Pts',(-2.82915649577662,-7.12325552842614,
11.5970972362655));
#42054=CARTESIAN_POINT('Ctrl Pts',(0.914441729670889,-7.60977608864241,
11.7159046174586));
#42055=CARTESIAN_POINT('Ctrl Pts',(4.43620077692759,-6.25020147401799,11.8347119986517));
#42056=CARTESIAN_POINT('Ctrl Pts',(6.8817587978778,-3.37435796188414,11.9535193798448));
#42057=CARTESIAN_POINT('Ctrl Pts',(7.6578351415651,0.320088602167681,12.072326761038));
#42058=CARTESIAN_POINT('Ctrl Pts',(6.57615742193745,3.93688321289441,12.1911341422311));
#42059=CARTESIAN_POINT('Ctrl Pts',(3.89913544126241,6.59860882907782,12.3099415234242));
#42060=CARTESIAN_POINT('Ctrl Pts',(0.276201937201886,7.65954361976593,12.4287489046173));
#42061=CARTESIAN_POINT('Ctrl Pts',(-3.41373689229886,6.86230982451555,12.5475562858105));
#42062=CARTESIAN_POINT('Ctrl Pts',(-6.27551940888551,4.40031267374749,12.6663636670036));
#42063=CARTESIAN_POINT('Ctrl Pts',(-7.61489125153754,0.870820600046571,
12.7851710481967));
#42064=CARTESIAN_POINT('Ctrl Pts',(-7.10692655121999,-2.86992802896064,
12.9039784293898));
#42065=CARTESIAN_POINT('Ctrl Pts',(-4.87485644851986,-5.91444656047583,
13.0227858105829));
#42066=CARTESIAN_POINT('Ctrl Pts',(-1.46016781772114,-7.52414740482518,
13.1415931917761));
#42067=CARTESIAN_POINT('Ctrl Pts',(2.30874711843974,-7.30852877128194,13.2604005729692));
#42068=CARTESIAN_POINT('Ctrl Pts',(5.51757774142707,-5.31989104535296,13.3792079541623));
#42069=CARTESIAN_POINT('Ctrl Pts',(7.38785742575197,-2.04068319962294,13.4980153353554));
#42070=CARTESIAN_POINT('Ctrl Pts',(7.46590388164774,1.73360404188074,13.6168227165485));
#42071=CARTESIAN_POINT('Ctrl Pts',(5.73270785128195,5.08728919315028,13.7356300977417));
#42072=CARTESIAN_POINT('Ctrl Pts',(2.60888235825391,7.20689693433218,13.8544374789348));
#42073=CARTESIAN_POINT('Ctrl Pts',(-1.14803759417921,7.57799995542215,13.9732448601279));
#42074=CARTESIAN_POINT('Ctrl Pts',(-4.62606968636267,6.11100406766213,14.092052241321));
#42075=CARTESIAN_POINT('Ctrl Pts',(-6.98261800673401,3.16092892461094,14.2108596225142));
#42076=CARTESIAN_POINT('Ctrl Pts',(-7.42306313170158,0.683868016819283,
14.2900645433096));
#42077=CARTESIAN_POINT('Ctrl Pts',(-7.33466990813749,-0.532853956222854,
14.3296670037073));
#42078=CARTESIAN_POINT('Ctrl Pts',(4.1021916212716,-5.75636310115763,-1.66533453693773E-15));
#42079=CARTESIAN_POINT('Ctrl Pts',(5.05709396285032,-5.0758653083813,0.0396024603977058));
#42080=CARTESIAN_POINT('Ctrl Pts',(6.62078237616492,-3.2312072264826,0.11880738119312));
#42081=CARTESIAN_POINT('Ctrl Pts',(7.35993086199691,0.321887848378951,0.237614762386243));
#42082=CARTESIAN_POINT('Ctrl Pts',(6.31364411820374,3.79596318205578,0.356422143579365));
#42083=CARTESIAN_POINT('Ctrl Pts',(3.73567782192208,6.34961322753113,0.475229524772488));
#42084=CARTESIAN_POINT('Ctrl Pts',(0.25146363409415,7.3626457790994,0.594036905965609));
#42085=CARTESIAN_POINT('Ctrl Pts',(-3.29375929907944,6.58965400328772,0.712844287158733));
#42086=CARTESIAN_POINT('Ctrl Pts',(-6.03992954092638,4.21798341238717,0.831651668351853));
#42087=CARTESIAN_POINT('Ctrl Pts',(-7.32084311808716,0.823081107049866,
0.950459049544977));
#42088=CARTESIAN_POINT('Ctrl Pts',(-6.8257546242272,-2.77151247120985,1.0692664307381));
#42089=CARTESIAN_POINT('Ctrl Pts',(-4.67477113205871,-5.69374237749066,
1.18807381193122));
#42090=CARTESIAN_POINT('Ctrl Pts',(-1.38971041869972,-7.23470180222814,
1.30688119312434));
#42091=CARTESIAN_POINT('Ctrl Pts',(2.23248728958399,-7.02055517652312,1.42568857431747));
#42092=CARTESIAN_POINT('Ctrl Pts',(5.31309433455675,-5.10325661323295,1.54449595551059));
#42093=CARTESIAN_POINT('Ctrl Pts',(7.10477015790912,-1.94793192835274,1.66330333670371));
#42094=CARTESIAN_POINT('Ctrl Pts',(7.17286283343114,1.67995141886001,1.78211071789683));
#42095=CARTESIAN_POINT('Ctrl Pts',(5.50085338730159,4.90028675314958,1.90091809908995));
#42096=CARTESIAN_POINT('Ctrl Pts',(2.49436329953803,6.93183595449864,2.01972548028308));
#42097=CARTESIAN_POINT('Ctrl Pts',(-1.1172473609771,7.28175504193768,2.1385328614762));
#42098=CARTESIAN_POINT('Ctrl Pts',(-4.45781917027722,5.86515526715037,2.25734024266932));
#42099=CARTESIAN_POINT('Ctrl Pts',(-6.71694543304686,3.02569696891267,2.37614762386244));
#42100=CARTESIAN_POINT('Ctrl Pts',(-7.34657295417076,-0.547780904931404,
2.49495500505557));
#42101=CARTESIAN_POINT('Ctrl Pts',(-6.19395711760227,-3.9883697563648,2.61376238624869));
#42102=CARTESIAN_POINT('Ctrl Pts',(-3.53871699613534,-6.46139923806788,
2.73256976744181));
#42103=CARTESIAN_POINT('Ctrl Pts',(-0.0250011063573954,-7.36692425873726,
2.85137714863493));
#42104=CARTESIAN_POINT('Ctrl Pts',(3.49477993190855,-6.48526879308302,2.97018452982806));
#42105=CARTESIAN_POINT('Ctrl Pts',(6.16674412284828,-4.03031822733696,3.08899191102118));
#42106=CARTESIAN_POINT('Ctrl Pts',(7.34268577093533,-0.597631792820449,
3.2077992922143));
#42107=CARTESIAN_POINT('Ctrl Pts',(6.73732707323029,2.98003724789039,3.32660667340742));
#42108=CARTESIAN_POINT('Ctrl Pts',(4.4975251459451,5.83476354722511,3.44541405460054));
#42109=CARTESIAN_POINT('Ctrl Pts',(1.16664519249845,7.27400419887887,3.56422143579367));
#42110=CARTESIAN_POINT('Ctrl Pts',(-2.44725728835037,6.94860632465767,3.68302881698679));
#42111=CARTESIAN_POINT('Ctrl Pts',(-5.46746689033045,4.93750988795068,3.80183619817991));
#42112=CARTESIAN_POINT('Ctrl Pts',(-7.16129525168959,1.72859723724002,3.92064357937304));
#42113=CARTESIAN_POINT('Ctrl Pts',(-7.11782773711273,-1.89966481129048,
4.03945096056615));
#42114=CARTESIAN_POINT('Ctrl Pts',(-5.34760935712609,-5.06707728913272,
4.15825834175928));
#42115=CARTESIAN_POINT('Ctrl Pts',(-2.28008659912764,-7.00524112296964,
4.2770657229524));
#42116=CARTESIAN_POINT('Ctrl Pts',(1.34057423043783,-7.24396706391966,4.39587310414552));
#42117=CARTESIAN_POINT('Ctrl Pts',(4.63601818231957,-5.72534134385619,4.51468048533865));
#42118=CARTESIAN_POINT('Ctrl Pts',(6.80678636175523,-2.81777527774835,4.63348786653177));
#42119=CARTESIAN_POINT('Ctrl Pts',(7.32626082140389,0.773369554113066,4.75229524772489));
#42120=CARTESIAN_POINT('Ctrl Pts',(6.06841954922959,4.17689864193457,4.87110262891801));
#42121=CARTESIAN_POINT('Ctrl Pts',(3.33840880410428,6.56713215545002,4.98991001011114));
#42122=CARTESIAN_POINT('Ctrl Pts',(-0.201483902833845,7.36421091002734,
5.10871739130425));
#42123=CARTESIAN_POINT('Ctrl Pts',(-3.69249758144563,6.37476742332494,5.22752477249739));
#42124=CARTESIAN_POINT('Ctrl Pts',(-6.28772905939532,3.83883593894067,5.34633215369049));
#42125=CARTESIAN_POINT('Ctrl Pts',(-7.35758762923681,0.371621270338646,
5.46513953488363));
#42126=CARTESIAN_POINT('Ctrl Pts',(-6.6425307339471,-3.18574693581189,5.58394691607674));
#42127=CARTESIAN_POINT('Ctrl Pts',(-4.3160277462564,-5.97026821709139,5.70275429726988));
#42128=CARTESIAN_POINT('Ctrl Pts',(-0.942477130941647,-7.30643106777301,
5.82156167846298));
#42129=CARTESIAN_POINT('Ctrl Pts',(2.659713915357,-6.87008878974086,5.94036905965612));
#42130=CARTESIAN_POINT('Ctrl Pts',(5.61667112421129,-4.76709592654876,6.05917644084923));
#42131=CARTESIAN_POINT('Ctrl Pts',(7.21105086102525,-1.50762845892934,6.17798382204236));
#42132=CARTESIAN_POINT('Ctrl Pts',(7.05606424975171,2.11758244086091,6.29679120323547));
#42133=CARTESIAN_POINT('Ctrl Pts',(5.18931029882807,5.22907799836104,6.41559858442861));
#42134=CARTESIAN_POINT('Ctrl Pts',(2.06365456208858,7.0720243169009,6.53440596562172));
#42135=CARTESIAN_POINT('Ctrl Pts',(-1.56263387223831,7.19933146005934,6.65321334681485));
#42136=CARTESIAN_POINT('Ctrl Pts',(-4.80983482498188,5.58011532558766,6.77202072800796));
#42137=CARTESIAN_POINT('Ctrl Pts',(-6.89019292155314,2.60718998046665,6.8908281092011));
#42138=CARTESIAN_POINT('Ctrl Pts',(-7.29902326702459,-0.998227147447127,
7.0096354903942));
#42139=CARTESIAN_POINT('Ctrl Pts',(-5.93714558070924,-4.36147915780088,
7.12844287158734));
#42140=CARTESIAN_POINT('Ctrl Pts',(-3.13494485649586,-6.66665724611644,
7.24725025278046));
#42141=CARTESIAN_POINT('Ctrl Pts',(0.427778451839743,-7.35453626591155,
7.36605763397357));
#42142=CARTESIAN_POINT('Ctrl Pts',(3.88672475977586,-6.25824006668105,7.48486501516671));
#42143=CARTESIAN_POINT('Ctrl Pts',(6.40277028527823,-3.64372484751866,7.60367239635982));
#42144=CARTESIAN_POINT('Ctrl Pts',(7.36553445311621,-0.145259458986194,
7.72247977755295));
#42145=CARTESIAN_POINT('Ctrl Pts',(6.54145529447003,3.38844517749906,7.84128715874606));
#42146=CARTESIAN_POINT('Ctrl Pts',(4.13045046018973,6.10012926800615,7.9600945399392));
#42147=CARTESIAN_POINT('Ctrl Pts',(0.71741815768671,7.33195125989582,8.0789019211323));
#42148=CARTESIAN_POINT('Ctrl Pts',(-2.86965634847726,6.78507704688097,8.19770930232544));
#42149=CARTESIAN_POINT('Ctrl Pts',(-5.76056598999791,4.59217568972987,8.31651668351855));
#42150=CARTESIAN_POINT('Ctrl Pts',(-7.25398995528984,1.28523453852627,8.43532406471168));
#42151=CARTESIAN_POINT('Ctrl Pts',(-6.98763075420087,-2.33349834656314,
8.55413144590481));
#42152=CARTESIAN_POINT('Ctrl Pts',(-5.02610585121275,-5.3861357263693,8.67293882709792));
#42153=CARTESIAN_POINT('Ctrl Pts',(-1.84527177852238,-7.1321224157929,8.79174620829105));
#42154=CARTESIAN_POINT('Ctrl Pts',(1.78321637602583,-7.14789041932932,8.91055358948417));
#42155=CARTESIAN_POINT('Ctrl Pts',(4.97910479168735,-5.42961449495844,9.02936097067729));
#42156=CARTESIAN_POINT('Ctrl Pts',(6.96708626922742,-2.39414013950925,9.14816835187041));
#42157=CARTESIAN_POINT('Ctrl Pts',(7.26488603837279,1.2221411292984,9.26697573306353));
#42158=CARTESIAN_POINT('Ctrl Pts',(5.80025930364893,4.54193682264524,9.38578311425666));
#42159=CARTESIAN_POINT('Ctrl Pts',(2.92851748521003,6.75988043010273,9.50459049544978));
#42160=CARTESIAN_POINT('Ctrl Pts',(-0.653668627291716,7.33790947178836,
9.6233978766429));
#42161=CARTESIAN_POINT('Ctrl Pts',(-4.07727786640525,6.1357968749453,9.74220525783602));
#42162=CARTESIAN_POINT('Ctrl Pts',(-6.51175905348377,3.44516938913589,9.86101263902915));
#42163=CARTESIAN_POINT('Ctrl Pts',(-7.36651873054104,-0.0812396642935325,
9.97982002022226));
#42164=CARTESIAN_POINT('Ctrl Pts',(-6.43419630013248,-3.58794036486512,
10.0986274014154));
#42165=CARTESIAN_POINT('Ctrl Pts',(-3.94096871160376,-6.22422394396494,
10.2174347826085));
#42166=CARTESIAN_POINT('Ctrl Pts',(-0.491681018131546,-7.35054065133146,
10.3362421638016));
#42167=CARTESIAN_POINT('Ctrl Pts',(3.07688613178757,-6.69365145660272,10.4550495449948));
#42168=CARTESIAN_POINT('Ctrl Pts',(5.8990154656956,-4.41291452737873,10.5738569261879));
#42169=CARTESIAN_POINT('Ctrl Pts',(7.2900719447016,-1.06162570218753,10.692664307381));
#42170=CARTESIAN_POINT('Ctrl Pts',(6.91259193977638,2.54720842582524,10.8114716885741));
#42171=CARTESIAN_POINT('Ctrl Pts',(4.85815028937904,5.53810200847668,10.9302790697673));
#42172=CARTESIAN_POINT('Ctrl Pts',(1.62514468290704,7.18547860967203,11.0490864509604));
#42173=CARTESIAN_POINT('Ctrl Pts',(-2.00211322794815,7.08969256829738,11.1678938321535));
#42174=CARTESIAN_POINT('Ctrl Pts',(-5.14366807368819,5.27398111849169,11.2867012133466));
#42175=CARTESIAN_POINT('Ctrl Pts',(-7.03739371845359,2.17882714820567,11.4055085945397));
#42176=CARTESIAN_POINT('Ctrl Pts',(-7.22388140497096,-1.44489983663997,
11.5243159757329));
#42177=CARTESIAN_POINT('Ctrl Pts',(-5.65789011484937,-4.71810105207384,
11.643123356926));
#42178=CARTESIAN_POINT('Ctrl Pts',(-2.71932182355139,-6.84671358480829,
11.7619307381191));
#42179=CARTESIAN_POINT('Ctrl Pts',(0.878940898310958,-7.31434624457016,
11.8807381193122));
#42180=CARTESIAN_POINT('Ctrl Pts',(4.26397677341757,-6.00755359247974,11.9995455005054));
#42181=CARTESIAN_POINT('Ctrl Pts',(6.61459233924385,-3.24335725504188,12.1183528816985));
#42182=CARTESIAN_POINT('Ctrl Pts',(7.36053952925658,0.307661991354685,12.2371602628916));
#42183=CARTESIAN_POINT('Ctrl Pts',(6.32085514508631,3.78404392036229,12.3559676440847));
#42184=CARTESIAN_POINT('Ctrl Pts',(3.74776160818102,6.3424349345032,12.4747750252778));
#42185=CARTESIAN_POINT('Ctrl Pts',(0.265479112470959,7.36218168021696,12.593582406471));
#42186=CARTESIAN_POINT('Ctrl Pts',(-3.28120740049152,6.59589842189123,12.7123897876641));
#42187=CARTESIAN_POINT('Ctrl Pts',(-6.03188862411031,4.22948193287789,12.8311971688572));
#42188=CARTESIAN_POINT('Ctrl Pts',(-7.31926282451633,0.837013246046923,
12.9500045500503));
#42189=CARTESIAN_POINT('Ctrl Pts',(-6.83101853784315,-2.75851050757525,
13.0688119312434));
#42190=CARTESIAN_POINT('Ctrl Pts',(-4.68560277486572,-5.6848334937073,13.1876193124366));
#42191=CARTESIAN_POINT('Ctrl Pts',(-1.40348058465622,-7.23204187258727,
13.3064266936297));
#42192=CARTESIAN_POINT('Ctrl Pts',(2.21911599220716,-7.02479407394702,13.4252340748228));
#42193=CARTESIAN_POINT('Ctrl Pts',(5.30337207849841,-5.11336005630641,13.5440414560159));
#42194=CARTESIAN_POINT('Ctrl Pts',(7.10104299890235,-1.96145896063838,13.6628488372091));
#42195=CARTESIAN_POINT('Ctrl Pts',(7.1760595033216,1.66630135572941,13.7816562184022));
#42196=CARTESIAN_POINT('Ctrl Pts',(5.51015031911699,4.88978836847741,13.9004635995953));
#42197=CARTESIAN_POINT('Ctrl Pts',(2.50759925881393,6.92710782979698,14.0192709807884));
#42198=CARTESIAN_POINT('Ctrl Pts',(-1.10346800849277,7.28380373740842,14.1380783619816));
#42199=CARTESIAN_POINT('Ctrl Pts',(-4.44647451428538,5.87376016484493,14.2568857431747));
#42200=CARTESIAN_POINT('Ctrl Pts',(-6.71153595058463,3.03821404726848,14.3756931243678));
#42201=CARTESIAN_POINT('Ctrl Pts',(-7.13488193451627,0.657318612576422,
14.4548980451632));
#42202=CARTESIAN_POINT('Ctrl Pts',(-7.04992034888086,-0.51216728169178,
14.4945005055609));
#42203=CARTESIAN_POINT('',(-7.90416902665076,-0.57422730528489,14.));
#42204=CARTESIAN_POINT('Ctrl Pts',(2.93403320825969,6.43108807842008,14.));
#42205=CARTESIAN_POINT('Ctrl Pts',(2.76504255556035,6.52067383231118,14.));
#42206=CARTESIAN_POINT('Ctrl Pts',(2.59273860581333,6.60318405968412,14.));
#42207=CARTESIAN_POINT('Ctrl Pts',(2.41754216546193,6.67839186611978,14.));
#42208=CARTESIAN_POINT('Ctrl Pts',(2.24288743377926,6.75336712947054,14.));
#42209=CARTESIAN_POINT('Ctrl Pts',(2.06535765963728,6.82108586425906,14.));
#42210=CARTESIAN_POINT('Ctrl Pts',(1.88543906684595,6.88157091887576,14.));
#42211=CARTESIAN_POINT('Ctrl Pts',(1.70341361000517,6.94276425930731,14.));
#42212=CARTESIAN_POINT('Ctrl Pts',(1.51894244701564,6.99655374698891,14.));
#42213=CARTESIAN_POINT('Ctrl Pts',(1.33250163756747,7.0429170614105,14.));
#42214=CARTESIAN_POINT('Ctrl Pts',(1.14527132784069,7.08947670543268,14.));
#42215=CARTESIAN_POINT('Ctrl Pts',(0.956053975526834,7.12854734578937,14.));
#42216=CARTESIAN_POINT('Ctrl Pts',(0.765314017071225,7.16005711178253,14.));
#42217=CARTESIAN_POINT('Ctrl Pts',(0.611878080828955,7.18540434623241,14.));
#42218=CARTESIAN_POINT('Ctrl Pts',(0.457456382235616,7.2058580443962,14.));
#42219=CARTESIAN_POINT('Ctrl Pts',(0.302286994143537,7.22135648777913,14.));
#42220=CARTESIAN_POINT('Ctrl Pts',(0.281945378131416,7.22338822475997,14.));
#42221=CARTESIAN_POINT('Ctrl Pts',(0.261593030742382,7.22533453564978,14.));
#42222=CARTESIAN_POINT('Ctrl Pts',(0.241239397075081,7.22719456829265,14.));
#42223=CARTESIAN_POINT('Ctrl Pts',(0.0463864417924064,7.24500135715949,
14.));
#42224=CARTESIAN_POINT('Ctrl Pts',(-0.148813863335687,7.25492811071152,
14.));
#42225=CARTESIAN_POINT('Ctrl Pts',(-0.343865896367492,7.25698779731808,
14.));
#42226=CARTESIAN_POINT('Ctrl Pts',(-0.540339607037362,7.25906249638231,
14.));
#42227=CARTESIAN_POINT('Ctrl Pts',(-0.736663568137468,7.25315522583491,
14.));
#42228=CARTESIAN_POINT('Ctrl Pts',(-0.93234903806384,7.23922981278962,14.));
#42229=CARTESIAN_POINT('Ctrl Pts',(-0.986489845986116,7.23537703254381,
14.));
#42230=CARTESIAN_POINT('Ctrl Pts',(-1.04058184869791,7.23091018259324,14.));
#42231=CARTESIAN_POINT('Ctrl Pts',(-1.09461482262646,7.22582780366122,14.));
#42232=CARTESIAN_POINT('Ctrl Pts',(-1.28889696859445,7.20755349051977,14.));
#42233=CARTESIAN_POINT('Ctrl Pts',(-1.48241602611913,7.18132540055054,14.));
#42234=CARTESIAN_POINT('Ctrl Pts',(-1.67474546639368,7.14734789612827,14.));
#42235=CARTESIAN_POINT('Ctrl Pts',(-1.86783518449381,7.11323607871085,14.));
#42236=CARTESIAN_POINT('Ctrl Pts',(-2.05972653856352,7.07131331315291,14.));
#42237=CARTESIAN_POINT('Ctrl Pts',(-2.24998149527249,7.02173429436054,14.));
#42238=CARTESIAN_POINT('Ctrl Pts',(-2.30504373785463,7.0073854857568,14.));
#42239=CARTESIAN_POINT('Ctrl Pts',(-2.35996883893649,6.99239506626978,14.));
#42240=CARTESIAN_POINT('Ctrl Pts',(-2.41474595378691,6.97676600288421,14.));
#42241=CARTESIAN_POINT('Ctrl Pts',(-2.44203939863075,6.96897860881207,14.));
#42242=CARTESIAN_POINT('Ctrl Pts',(-2.46929610147469,6.96103265538078,14.));
#42243=CARTESIAN_POINT('Ctrl Pts',(-2.49651470828259,6.95292847781968,14.));
#42244=CARTESIAN_POINT('Ctrl Pts',(-2.51941719524455,6.94610939915631,14.));
#42245=CARTESIAN_POINT('Ctrl Pts',(-2.54229321057616,6.93917809579522,14.));
#42246=CARTESIAN_POINT('Ctrl Pts',(-2.56512697365784,6.93213951209675,14.));
#42247=CARTESIAN_POINT('Ctrl Pts',(-2.7549248933863,6.87363366971651,14.));
#42248=CARTESIAN_POINT('Ctrl Pts',(-2.94205306639717,6.80764665211765,14.));
#42249=CARTESIAN_POINT('Ctrl Pts',(-3.12608192497131,6.73444312052763,14.));
#42250=CARTESIAN_POINT('Ctrl Pts',(-3.31147248647493,6.66069792680816,14.));
#42251=CARTESIAN_POINT('Ctrl Pts',(-3.49371837629268,6.57962887889023,14.));
#42252=CARTESIAN_POINT('Ctrl Pts',(-3.67237779134679,6.49145335616022,14.));
#42253=CARTESIAN_POINT('Ctrl Pts',(-3.85086973913998,6.40336048518,14.));
#42254=CARTESIAN_POINT('Ctrl Pts',(-4.02578261635796,6.30817424132695,14.));
#42255=CARTESIAN_POINT('Ctrl Pts',(-4.19666301580165,6.20606133279816,14.));
#42256=CARTESIAN_POINT('Ctrl Pts',(-4.31144240408791,6.13747267537916,14.));
#42257=CARTESIAN_POINT('Ctrl Pts',(-4.42440217223988,6.06575786401773,14.));
#42258=CARTESIAN_POINT('Ctrl Pts',(-4.53539929999993,5.99095543969761,14.));
#42259=CARTESIAN_POINT('Ctrl Pts',(-4.6664170622633,5.90266084645836,14.));
#42260=CARTESIAN_POINT('Ctrl Pts',(-4.79470072581212,5.81006464588512,14.));
#42261=CARTESIAN_POINT('Ctrl Pts',(-4.92009686878172,5.71333951420776,14.));
#42262=CARTESIAN_POINT('Ctrl Pts',(-4.94938301419314,5.69074945518235,14.));
#42263=CARTESIAN_POINT('Ctrl Pts',(-4.97851160360603,5.66793411403788,14.));
#42264=CARTESIAN_POINT('Ctrl Pts',(-5.00748057682806,5.64489556783237,14.));
#42265=CARTESIAN_POINT('Ctrl Pts',(-5.02640283917017,5.62984700494612,14.));
#42266=CARTESIAN_POINT('Ctrl Pts',(-5.0452569991305,5.614703208918,14.));
#42267=CARTESIAN_POINT('Ctrl Pts',(-5.06404247259783,5.5994647485729,14.));
#42268=CARTESIAN_POINT('Ctrl Pts',(-5.0845422812029,5.58283564837728,14.));
#42269=CARTESIAN_POINT('Ctrl Pts',(-5.10495401158589,5.56609887849884,14.));
#42270=CARTESIAN_POINT('Ctrl Pts',(-5.12527090278503,5.54926057344536,14.));
#42271=CARTESIAN_POINT('Ctrl Pts',(-5.27876145036398,5.42205013373652,14.));
#42272=CARTESIAN_POINT('Ctrl Pts',(-5.42695161912127,5.28895862038518,14.));
#42273=CARTESIAN_POINT('Ctrl Pts',(-5.56960113735066,5.15042741208114,14.));
#42274=CARTESIAN_POINT('Ctrl Pts',(-5.71675997622002,5.00751706780356,14.));
#42275=CARTESIAN_POINT('Ctrl Pts',(-5.85802295965456,4.85881742447612,14.));
#42276=CARTESIAN_POINT('Ctrl Pts',(-5.99310134761184,4.70476219817552,14.));
#42277=CARTESIAN_POINT('Ctrl Pts',(-6.12679686666241,4.55228411671349,14.));
#42278=CARTESIAN_POINT('Ctrl Pts',(-6.25443422790721,4.39455895812829,14.));
#42279=CARTESIAN_POINT('Ctrl Pts',(-6.37570151960029,4.2319651250009,14.));
#42280=CARTESIAN_POINT('Ctrl Pts',(-6.49885028909018,4.06684862741341,14.));
#42281=CARTESIAN_POINT('Ctrl Pts',(-6.6154304429211,3.89671076483844,14.));
#42282=CARTESIAN_POINT('Ctrl Pts',(-6.72507364482188,3.72191167969025,14.));
#42283=CARTESIAN_POINT('Ctrl Pts',(-6.77989524577227,3.63451213711615,14.));
#42284=CARTESIAN_POINT('Ctrl Pts',(-6.8329819009625,3.54594677032576,14.));
#42285=CARTESIAN_POINT('Ctrl Pts',(-6.88428295688164,3.45625783325501,14.));
#42286=CARTESIAN_POINT('Ctrl Pts',(-6.90360298603292,3.42248088953117,14.));
#42287=CARTESIAN_POINT('Ctrl Pts',(-6.9226697332359,3.38854457515301,14.));
#42288=CARTESIAN_POINT('Ctrl Pts',(-6.94148036875173,3.35445108984207,14.));
#42289=CARTESIAN_POINT('Ctrl Pts',(-6.95472025012042,3.33045436200255,14.));
#42290=CARTESIAN_POINT('Ctrl Pts',(-6.96783370790352,3.30637881270687,14.));
#42291=CARTESIAN_POINT('Ctrl Pts',(-6.98081173224686,3.28224040555493,14.));
#42292=CARTESIAN_POINT('Ctrl Pts',(-6.99835567955093,3.24960963434707,14.));
#42293=CARTESIAN_POINT('Ctrl Pts',(-7.01565566297557,3.2168576748347,14.));
#42294=CARTESIAN_POINT('Ctrl Pts',(-7.03270997223139,3.18398692053127,14.));
#42295=CARTESIAN_POINT('Ctrl Pts',(-7.12613862865058,3.00391100165421,14.));
#42296=CARTESIAN_POINT('Ctrl Pts',(-7.21219748995004,2.82027261069025,14.));
#42297=CARTESIAN_POINT('Ctrl Pts',(-7.29087218921779,2.63356828668566,14.));
#42298=CARTESIAN_POINT('Ctrl Pts',(-7.37042005988303,2.44479182415336,14.));
#42299=CARTESIAN_POINT('Ctrl Pts',(-7.44241921699479,2.25288041051982,14.));
#42300=CARTESIAN_POINT('Ctrl Pts',(-7.50681051535069,2.05831727163918,14.));
#42301=CARTESIAN_POINT('Ctrl Pts',(-7.54180528095381,1.95257796191906,14.));
#42302=CARTESIAN_POINT('Ctrl Pts',(-7.57455220017289,1.84605497185642,14.));
#42303=CARTESIAN_POINT('Ctrl Pts',(-7.60503595657932,1.73882316930943,14.));
#42304=CARTESIAN_POINT('Ctrl Pts',(-7.62917933121202,1.65389473900327,14.));
#42305=CARTESIAN_POINT('Ctrl Pts',(-7.65190299831561,1.56852164701574,14.));
#42306=CARTESIAN_POINT('Ctrl Pts',(-7.6731974479298,1.48274048861856,14.));
#42307=CARTESIAN_POINT('Ctrl Pts',(-7.68040437951521,1.45370856006032,14.));
#42308=CARTESIAN_POINT('Ctrl Pts',(-7.68744763881537,1.42462944784155,14.));
#42309=CARTESIAN_POINT('Ctrl Pts',(-7.69432342715027,1.39551958977078,14.));
#42310=CARTESIAN_POINT('Ctrl Pts',(-7.74209559420721,1.19326772641705,14.));
#42311=CARTESIAN_POINT('Ctrl Pts',(-7.78183126083143,0.989359506012121,
14.));
#42312=CARTESIAN_POINT('Ctrl Pts',(-7.81348695611449,0.784295778626206,
14.));
#42313=CARTESIAN_POINT('Ctrl Pts',(-7.84522934883263,0.578670430368129,
14.));
#42314=CARTESIAN_POINT('Ctrl Pts',(-7.86884766179871,0.371882565380943,
14.));
#42315=CARTESIAN_POINT('Ctrl Pts',(-7.88424943003973,0.164417795820874,
14.));
#42316=CARTESIAN_POINT('Ctrl Pts',(-7.89954884786313,-0.0416682940011354,
14.));
#42317=CARTESIAN_POINT('Ctrl Pts',(-7.90674070299934,-0.248423003209867,
14.));
#42318=CARTESIAN_POINT('Ctrl Pts',(-7.90568392850165,-0.455379271744865,
14.));
#42319=CARTESIAN_POINT('Ctrl Pts',(-7.90548167065186,-0.494988980311862,
14.));
#42320=CARTESIAN_POINT('Ctrl Pts',(-7.90497710617671,-0.534606081175834,
14.));
#42321=CARTESIAN_POINT('Ctrl Pts',(-7.90416902665075,-0.574227305285002,
14.));
#42322=CARTESIAN_POINT('Ctrl Pts',(3.45507168555155,7.13251860299055,1.38777878078145E-16));
#42323=CARTESIAN_POINT('Ctrl Pts',(3.6420087970317,7.02984949182691,9.74215697402965E-17));
#42324=CARTESIAN_POINT('Ctrl Pts',(3.82450583053849,6.9197446466761,9.77074144499948E-16));
#42325=CARTESIAN_POINT('Ctrl Pts',(4.00206481978707,6.8023508547206,7.66747776381749E-16));
#42326=CARTESIAN_POINT('Ctrl Pts',(4.17547768173782,6.68769829038464,5.61332676907285E-16));
#42327=CARTESIAN_POINT('Ctrl Pts',(4.34418082373008,6.56609255773603,6.25535711258445E-17));
#42328=CARTESIAN_POINT('Ctrl Pts',(4.50784061150571,6.43790653945084,1.11022302462516E-16));
#42329=CARTESIAN_POINT('Ctrl Pts',(4.61464463848975,6.3542526184603,1.42652892724929E-16));
#42330=CARTESIAN_POINT('Ctrl Pts',(4.71930009693716,6.26779542334385,5.52961652623665E-16));
#42331=CARTESIAN_POINT('Ctrl Pts',(4.82170530078264,6.17863067064047,5.27355936696949E-16));
#42332=CARTESIAN_POINT('Ctrl Pts',(4.88074840962393,6.12722152343917,5.12592613978494E-16));
#42333=CARTESIAN_POINT('Ctrl Pts',(4.93904333883909,6.07491220743105,5.36534324121204E-16));
#42334=CARTESIAN_POINT('Ctrl Pts',(4.99656940254868,6.02172027598176,4.78783679369599E-16));
#42335=CARTESIAN_POINT('Ctrl Pts',(5.02400664443905,5.99635021247181,4.51239322825865E-16));
#42336=CARTESIAN_POINT('Ctrl Pts',(5.05126896812563,5.97077935983458,2.70409761827241E-16));
#42337=CARTESIAN_POINT('Ctrl Pts',(5.0783540546327,5.94500958145069,2.70616862252382E-16));
#42338=CARTESIAN_POINT('Ctrl Pts',(5.09938650653718,5.92499850914687,2.70777682478303E-16));
#42339=CARTESIAN_POINT('Ctrl Pts',(5.12031166695779,5.90486781053517,5.18028363593499E-16));
#42340=CARTESIAN_POINT('Ctrl Pts',(5.14111885655612,5.88462789262779,5.27355936696949E-16));
#42341=CARTESIAN_POINT('Ctrl Pts',(5.28891173105196,5.74086433277962,5.93609422518019E-16));
#42342=CARTESIAN_POINT('Ctrl Pts',(5.43088438187667,5.59147180641874,1.17436207753861E-15));
#42343=CARTESIAN_POINT('Ctrl Pts',(5.56671584293328,5.43681933615198,1.12410081243297E-15));
#42344=CARTESIAN_POINT('Ctrl Pts',(5.70192563898127,5.28287466972178,1.07406957996898E-15));
#42345=CARTESIAN_POINT('Ctrl Pts',(5.83105073149007,5.12371752674162,1.15095222081023E-15));
#42346=CARTESIAN_POINT('Ctrl Pts',(5.95373293436354,4.95968187186966,1.16573417585641E-15));
#42347=CARTESIAN_POINT('Ctrl Pts',(6.07188941364143,4.80169746172905,1.17997082733635E-15));
#42348=CARTESIAN_POINT('Ctrl Pts',(6.18406970280772,4.63918724659927,6.53710017676321E-16));
#42349=CARTESIAN_POINT('Ctrl Pts',(6.2899117761523,4.47243030721014,6.38378239159465E-16));
#42350=CARTESIAN_POINT('Ctrl Pts',(6.30776551361993,4.44430127947401,6.35792031804469E-16));
#42351=CARTESIAN_POINT('Ctrl Pts',(6.32543880171542,4.41605138142731,4.74985180111043E-16));
#42352=CARTESIAN_POINT('Ctrl Pts',(6.34292977552621,4.38768191358574,4.71844785465692E-16));
#42353=CARTESIAN_POINT('Ctrl Pts',(6.35742061123199,4.36417851680525,4.69243046800403E-16));
#42354=CARTESIAN_POINT('Ctrl Pts',(6.37178685416811,4.34059204937566,4.85771739497528E-16));
#42355=CARTESIAN_POINT('Ctrl Pts',(6.3860185636023,4.31693826780559,4.71844785465692E-16));
#42356=CARTESIAN_POINT('Ctrl Pts',(6.45644594201099,4.19988459739906,4.02925526945434E-16));
#42357=CARTESIAN_POINT('Ctrl Pts',(6.52363145866076,4.08109952203915,7.5220568606171E-16));
#42358=CARTESIAN_POINT('Ctrl Pts',(6.5874832695581,3.96068897350107,6.93889390390723E-16));
#42359=CARTESIAN_POINT('Ctrl Pts',(6.68217425780676,3.7821224821769,6.06284321176324E-16));
#42360=CARTESIAN_POINT('Ctrl Pts',(6.76953599931651,3.59998206678033,1.56378908891375E-15));
#42361=CARTESIAN_POINT('Ctrl Pts',(6.84949791164232,3.414750736673,1.41553435639707E-15));
#42362=CARTESIAN_POINT('Ctrl Pts',(6.92987732361558,3.22855227092865,1.26650555161578E-15));
#42363=CARTESIAN_POINT('Ctrl Pts',(7.00277959908613,3.0392298331746,8.2787151976317E-16));
#42364=CARTESIAN_POINT('Ctrl Pts',(7.06808334347011,2.84725669514074,9.15933995315754E-16));
#42365=CARTESIAN_POINT('Ctrl Pts',(7.13316081883727,2.65594871916779,1.00369134579549E-15));
#42366=CARTESIAN_POINT('Ctrl Pts',(7.19069243071623,2.46200767909707,3.56302599425838E-16));
#42367=CARTESIAN_POINT('Ctrl Pts',(7.24050690007108,2.26589526878088,1.94289029309402E-16));
#42368=CARTESIAN_POINT('Ctrl Pts',(7.28067447006557,2.10776131553028,6.36504517637552E-17));
#42369=CARTESIAN_POINT('Ctrl Pts',(7.315823496763,1.94821528841226,8.453426307217E-16));
#42370=CARTESIAN_POINT('Ctrl Pts',(7.34583909427119,1.78750071388778,9.71445146547012E-16));
#42371=CARTESIAN_POINT('Ctrl Pts',(7.35704804173394,1.72748387691319,1.0185365454246E-15));
#42372=CARTESIAN_POINT('Ctrl Pts',(7.3675408759556,1.66730411324232,2.17326548184769E-16));
#42373=CARTESIAN_POINT('Ctrl Pts',(7.37731078948879,1.60697426365927,1.94289029309402E-16));
#42374=CARTESIAN_POINT('Ctrl Pts',(7.38106886176767,1.5837679236506,1.85427470733132E-16));
#42375=CARTESIAN_POINT('Ctrl Pts',(7.38471928344393,1.56054340131122,4.77709052170576E-16));
#42376=CARTESIAN_POINT('Ctrl Pts',(7.38826041896046,1.53731084403494,4.71844785465692E-16));
#42377=CARTESIAN_POINT('Ctrl Pts',(7.41886472277194,1.3365232046228,4.2116279404502E-16));
#42378=CARTESIAN_POINT('Ctrl Pts',(7.44134458470096,1.13492783993692,6.75143946583213E-16));
#42379=CARTESIAN_POINT('Ctrl Pts',(7.45560296537357,0.933000562371476,6.66133814775094E-16));
#42380=CARTESIAN_POINT('Ctrl Pts',(7.46986134604617,0.73107328480603,6.57123682966975E-16));
#42381=CARTESIAN_POINT('Ctrl Pts',(7.47589835898452,0.528813351042067,7.55757054193326E-16));
#42382=CARTESIAN_POINT('Ctrl Pts',(7.47356156794063,0.326692878441132,7.7715611723761E-16));
#42383=CARTESIAN_POINT('Ctrl Pts',(7.47125585823871,0.127260782939089,7.97159268077648E-16));
#42384=CARTESIAN_POINT('Ctrl Pts',(7.46079730105774,-0.0720362355310806,
1.05905070470954E-15));
#42385=CARTESIAN_POINT('Ctrl Pts',(7.44230228855497,-0.27072027972702,1.16573417585641E-15));
#42386=CARTESIAN_POINT('Ctrl Pts',(7.42387912549052,-0.468632476000395,
1.27200320297528E-15));
#42387=CARTESIAN_POINT('Ctrl Pts',(7.39748157902158,-0.665937128618222,
5.79302131420473E-16));
#42388=CARTESIAN_POINT('Ctrl Pts',(7.36317622914462,-0.862144580575266,
4.9960036108132E-16));
#42389=CARTESIAN_POINT('Ctrl Pts',(7.34534425788565,-0.964133502321923,
4.58171263780931E-16));
#42390=CARTESIAN_POINT('Ctrl Pts',(7.32537487422037,-1.06582562028994,7.21644966006352E-16));
#42391=CARTESIAN_POINT('Ctrl Pts',(7.30327255511682,-1.16714938005994,7.21644966006352E-16));
#42392=CARTESIAN_POINT('Ctrl Pts',(7.29547904052248,-1.20287722367765,7.21644966006352E-16));
#42393=CARTESIAN_POINT('Ctrl Pts',(7.28742029945016,-1.2385592476155,1.5456272759111E-16));
#42394=CARTESIAN_POINT('Ctrl Pts',(7.27909643303922,-1.27419224578704,1.66533453693773E-16));
#42395=CARTESIAN_POINT('Ctrl Pts',(7.27441311892008,-1.29424068424165,1.73268625524415E-16));
#42396=CARTESIAN_POINT('Ctrl Pts',(7.26964620235591,-1.31427208877122,4.46372318945195E-16));
#42397=CARTESIAN_POINT('Ctrl Pts',(7.2647980511884,-1.33427665732707,4.44089209850063E-16));
#42398=CARTESIAN_POINT('Ctrl Pts',(7.21840223365521,-1.52571629699151,4.22240321619022E-16));
#42399=CARTESIAN_POINT('Ctrl Pts',(7.16451638886665,-1.7149352220374,3.12106949810161E-16));
#42400=CARTESIAN_POINT('Ctrl Pts',(7.10329533865964,-1.90148669058875,3.88578058618805E-16));
#42401=CARTESIAN_POINT('Ctrl Pts',(7.04213056723852,-2.08786666763316,4.64978869692518E-16));
#42402=CARTESIAN_POINT('Ctrl Pts',(6.97364382047475,-2.27158476110692,9.69884134728085E-16));
#42403=CARTESIAN_POINT('Ctrl Pts',(6.89794024185636,-2.45217911765423,9.43689570931383E-16));
#42404=CARTESIAN_POINT('Ctrl Pts',(6.82314219117491,-2.63061329580456,9.17808333264654E-16));
#42405=CARTESIAN_POINT('Ctrl Pts',(6.74129861780265,-2.80599860597599,9.09181254042411E-16));
#42406=CARTESIAN_POINT('Ctrl Pts',(6.65246709843858,-2.97786432931071,9.43689570931383E-16));
#42407=CARTESIAN_POINT('Ctrl Pts',(6.61552124306282,-3.04934488265293,9.58041900984587E-16));
#42408=CARTESIAN_POINT('Ctrl Pts',(6.57736610796479,-3.12021626253885,5.33583017232773E-16));
#42409=CARTESIAN_POINT('Ctrl Pts',(6.53800374880911,-3.19044292966702,5.55111512312578E-16));
#42410=CARTESIAN_POINT('Ctrl Pts',(6.46524483331982,-3.32025263234427,5.91589444244136E-16));
#42411=CARTESIAN_POINT('Ctrl Pts',(6.3883617494256,-3.44786031881024,-2.27018868370244E-16));
#42412=CARTESIAN_POINT('Ctrl Pts',(6.30748276302585,-3.57309566094206,-2.22044604925031E-16));
#42413=CARTESIAN_POINT('Ctrl Pts',(6.27209820647596,-3.62788612312473,-2.19868364667751E-16));
#42414=CARTESIAN_POINT('Ctrl Pts',(6.23594866787022,-3.6822223312132,-3.68266482884187E-16));
#42415=CARTESIAN_POINT('Ctrl Pts',(6.19904427211388,-3.73608917380381,-3.88578058618805E-16));
#42416=CARTESIAN_POINT('Ctrl Pts',(6.17970531144325,-3.76431694258207,-3.9922190622124E-16));
#42417=CARTESIAN_POINT('Ctrl Pts',(6.16015905662018,-3.79241581180823,5.43707389881397E-16));
#42418=CARTESIAN_POINT('Ctrl Pts',(6.14040692779842,-3.82038354608065,5.55111512312578E-16));
#42419=CARTESIAN_POINT('Ctrl Pts',(6.12153607086139,-3.8471034564797,5.66006822121118E-16));
#42420=CARTESIAN_POINT('Ctrl Pts',(6.10247388896415,-3.87370824653046,1.02099134177972E-15));
#42421=CARTESIAN_POINT('Ctrl Pts',(6.08324096182102,-3.90016965047398,9.99200722162641E-16));
#42422=CARTESIAN_POINT('Ctrl Pts',(5.96996686583548,-4.05601652640207,8.708628607586E-16));
#42423=CARTESIAN_POINT('Ctrl Pts',(5.8506722262936,-4.20704035147389,-2.21077044790491E-16));
#42424=CARTESIAN_POINT('Ctrl Pts',(5.72571543255065,-4.35294139755716,-1.66533453693773E-16));
#42425=CARTESIAN_POINT('Ctrl Pts',(5.60007830524651,-4.49963680923906,-1.11692897266405E-16));
#42426=CARTESIAN_POINT('Ctrl Pts',(5.46871669315143,-4.6411540157118,-4.73134212314551E-17));
#42427=CARTESIAN_POINT('Ctrl Pts',(5.33195525691958,-4.77715417893452,0.));
#42428=CARTESIAN_POINT('Ctrl Pts',(5.19597017321587,-4.91238231114137,4.70448375195555E-17));
#42429=CARTESIAN_POINT('Ctrl Pts',(5.0546458490692,-5.04215629186066,2.36926123753037E-16));
#42430=CARTESIAN_POINT('Ctrl Pts',(4.90827039206033,-5.16610237423274,2.77555756156289E-16));
#42431=CARTESIAN_POINT('Ctrl Pts',(4.76469954653324,-5.28767360078646,3.17406908779753E-16));
#42432=CARTESIAN_POINT('Ctrl Pts',(4.61626873550147,-5.40363841496088,-2.02048309080252E-16));
#42433=CARTESIAN_POINT('Ctrl Pts',(4.46322798222506,-5.51359971846396,-2.77555756156289E-16));
#42434=CARTESIAN_POINT('Ctrl Pts',(4.34557184220504,-5.59813682537676,-3.35605096449897E-16));
#42435=CARTESIAN_POINT('Ctrl Pts',(4.22519056171548,-5.67912480220418,7.48609313291272E-17));
#42436=CARTESIAN_POINT('Ctrl Pts',(4.10219162127164,-5.7563631011576,5.55111512312578E-17));
#42437=CARTESIAN_POINT('Ctrl Pts',(-7.90416902665075,-0.574227305285002,
14.));
#42438=CARTESIAN_POINT('Ctrl Pts',(-7.91805025518235,-0.383153882615103,
13.9942289417884));
#42439=CARTESIAN_POINT('Ctrl Pts',(-7.92486895290159,-0.191581382856594,
13.9884578835768));
#42440=CARTESIAN_POINT('Ctrl Pts',(-7.92471172241511,-8.01339879119567E-6,
13.9826868253652));
#42441=CARTESIAN_POINT('Origin',(0.,0.,0.));
#42442=CARTESIAN_POINT('Origin',(0.,0.,14.));
#42443=CARTESIAN_POINT('Origin',(0.,0.,-8.));
#42444=CARTESIAN_POINT('',(-7.,-8.57252759403147E-16,-8.));
#42445=CARTESIAN_POINT('Origin',(0.,0.,-8.));
#42446=CARTESIAN_POINT('',(-6.,-7.34788079488412E-16,-8.));
#42447=CARTESIAN_POINT('Origin',(0.,0.,-8.));
#42448=CARTESIAN_POINT('Origin',(0.,0.,-10.));
#42449=CARTESIAN_POINT('',(-7.,-8.57252759403147E-16,-10.));
#42450=CARTESIAN_POINT('Origin',(0.,0.,-10.));
#42451=CARTESIAN_POINT('',(-6.,7.34788079488412E-16,-10.));
#42452=CARTESIAN_POINT('Origin',(0.,0.,-10.));
#42453=CARTESIAN_POINT('Origin',(0.,0.,-10.));
#42454=CARTESIAN_POINT('',(-7.,-8.57252759403147E-16,-10.));
#42455=CARTESIAN_POINT('Origin',(0.,0.,-26.));
#42456=CARTESIAN_POINT('',(-6.,-7.34788079488412E-16,-14.));
#42457=CARTESIAN_POINT('',(-6.,-7.34788079488412E-16,-26.));
#42458=CARTESIAN_POINT('Origin',(0.,0.,-14.));
#42459=CARTESIAN_POINT('Origin',(0.,0.,-14.));
#42460=CARTESIAN_POINT('',(-7.,-8.57252759403147E-16,-14.));
#42461=CARTESIAN_POINT('Origin',(0.,0.,-14.));
#42462=CARTESIAN_POINT('Origin',(0.,0.,-16.));
#42463=CARTESIAN_POINT('',(-7.,-8.57252759403147E-16,-16.));
#42464=CARTESIAN_POINT('Origin',(0.,0.,-16.));
#42465=CARTESIAN_POINT('',(-6.,7.34788079488412E-16,-16.));
#42466=CARTESIAN_POINT('Origin',(0.,0.,-16.));
#42467=CARTESIAN_POINT('Origin',(0.,0.,-16.));
#42468=CARTESIAN_POINT('',(-7.,-8.57252759403147E-16,-16.));
#42469=CARTESIAN_POINT('Origin',(0.,0.,-26.));
#42470=CARTESIAN_POINT('',(-6.,-7.34788079488412E-16,-20.));
#42471=CARTESIAN_POINT('',(-6.,-7.34788079488412E-16,-26.));
#42472=CARTESIAN_POINT('Origin',(0.,0.,-20.));
#42473=CARTESIAN_POINT('Origin',(0.,0.,-20.));
#42474=CARTESIAN_POINT('',(-7.,-8.57252759403147E-16,-20.));
#42475=CARTESIAN_POINT('Origin',(0.,0.,-20.));
#42476=CARTESIAN_POINT('Origin',(0.,0.,-22.));
#42477=CARTESIAN_POINT('',(-7.,-8.57252759403147E-16,-22.));
#42478=CARTESIAN_POINT('Origin',(0.,0.,-22.));
#42479=CARTESIAN_POINT('',(-6.,7.34788079488412E-16,-22.));
#42480=CARTESIAN_POINT('Origin',(0.,0.,-22.));
#42481=CARTESIAN_POINT('Origin',(0.,0.,-22.));
#42482=CARTESIAN_POINT('',(-7.,-8.57252759403147E-16,-22.));
#42483=CARTESIAN_POINT('Origin',(0.,0.,-26.));
#42484=CARTESIAN_POINT('',(-6.,-7.34788079488412E-16,-26.));
#42485=CARTESIAN_POINT('',(-6.,-7.34788079488412E-16,-26.));
#42486=CARTESIAN_POINT('Origin',(0.,0.,-26.));
#42487=CARTESIAN_POINT('Origin',(0.,0.,-26.));
#42488=CARTESIAN_POINT('',(-6.,-7.34788079488412E-16,-6.));
#42489=CARTESIAN_POINT('Origin',(0.,0.,-6.));
#42490=CARTESIAN_POINT('',(-6.,-7.34788079488412E-16,-26.));
#42491=CARTESIAN_POINT('Origin',(0.,0.,-26.));
#42492=CARTESIAN_POINT('',(-4.,-4.89858719658941E-16,-26.));
#42493=CARTESIAN_POINT('Origin',(0.,0.,-26.));
#42494=CARTESIAN_POINT('Origin',(0.,0.,0.));
#42495=CARTESIAN_POINT('',(-12.,-1.46957615897682E-15,0.));
#42496=CARTESIAN_POINT('Origin',(0.,0.,0.));
#42497=CARTESIAN_POINT('Origin',(0.,0.,-6.));
#42498=CARTESIAN_POINT('',(-12.,-1.46957615897682E-15,-6.));
#42499=CARTESIAN_POINT('',(-12.,-1.46957615897682E-15,-6.));
#42500=CARTESIAN_POINT('Origin',(0.,0.,-6.));
#42501=CARTESIAN_POINT('Origin',(0.,0.,-6.));
#42502=CARTESIAN_POINT('Origin',(0.,0.,0.));
#42503=CARTESIAN_POINT('',(-4.,-4.89858719658941E-16,14.));
#42504=CARTESIAN_POINT('Origin',(0.,0.,14.));
#42505=CARTESIAN_POINT('',(-4.,-4.89858719658941E-16,0.));
#42506=CARTESIAN_POINT('Origin',(0.,0.,14.));
#42606=UNCERTAINTY_MEASURE_WITH_UNIT(LENGTH_MEASURE(0.01),#42621,
'DISTANCE_ACCURACY_VALUE',
'Maximum model space distance between geometric entities at asserted c
onnectivities');
#42608=UNCERTAINTY_MEASURE_WITH_UNIT(LENGTH_MEASURE(0.01),#42621,
'DISTANCE_ACCURACY_VALUE',
'Maximum model space distance between geometric entities at asserted c
onnectivities');
#42618=(
GEOMETRIC_REPRESENTATION_CONTEXT(3)
GLOBAL_UNCERTAINTY_ASSIGNED_CONTEXT((#42606))
GLOBAL_UNIT_ASSIGNED_CONTEXT((#42621,#42623,#42624))
REPRESENTATION_CONTEXT('','3D')
);
#42620=(
GEOMETRIC_REPRESENTATION_CONTEXT(3)
GLOBAL_UNCERTAINTY_ASSIGNED_CONTEXT((#42608))
GLOBAL_UNIT_ASSIGNED_CONTEXT((#42621,#42623,#42624))
REPRESENTATION_CONTEXT('','3D')
);
#42621=(
LENGTH_UNIT()
NAMED_UNIT(*)
SI_UNIT(.MILLI.,.METRE.)
);
#42623=(
NAMED_UNIT(*)
PLANE_ANGLE_UNIT()
SI_UNIT($,.RADIAN.)
);
#42624=(
NAMED_UNIT(*)
SI_UNIT($,.STERADIAN.)
SOLID_ANGLE_UNIT()
);
#42634=SHAPE_DEFINITION_REPRESENTATION(#42645,#42731);
#42645=PRODUCT_DEFINITION_SHAPE('',$,#42743);
#42731=SHAPE_REPRESENTATION('',(#11159),#42618);
#42733=PRODUCT_DEFINITION_CONTEXT('part definition',#42768,'design');
#42743=PRODUCT_DEFINITION('Hose connection','Hose connection',#42754,#42733);
#42754=PRODUCT_DEFINITION_FORMATION('',$,#42779);
#42768=APPLICATION_CONTEXT(
'Core Data for Automotive Mechanical Design Process');
#42769=PRODUCT_CONTEXT('part definition',#42768,'mechanical');
#42779=PRODUCT('Hose connection','Hose connection',$,(#42769));
#42787=PRESENTATION_STYLE_ASSIGNMENT((#42795));
#42795=SURFACE_STYLE_USAGE(.BOTH.,#42803);
#42803=SURFACE_SIDE_STYLE('',(#42811));
#42811=SURFACE_STYLE_FILL_AREA(#42819);
#42819=FILL_AREA_STYLE('Gray',(#42827));
#42827=FILL_AREA_STYLE_COLOUR('Gray',#42835);
#42835=COLOUR_RGB('Gray',0.407843137254902,0.447058823529412,0.498039215686275);
ENDSEC;
END-ISO-10303-21;
